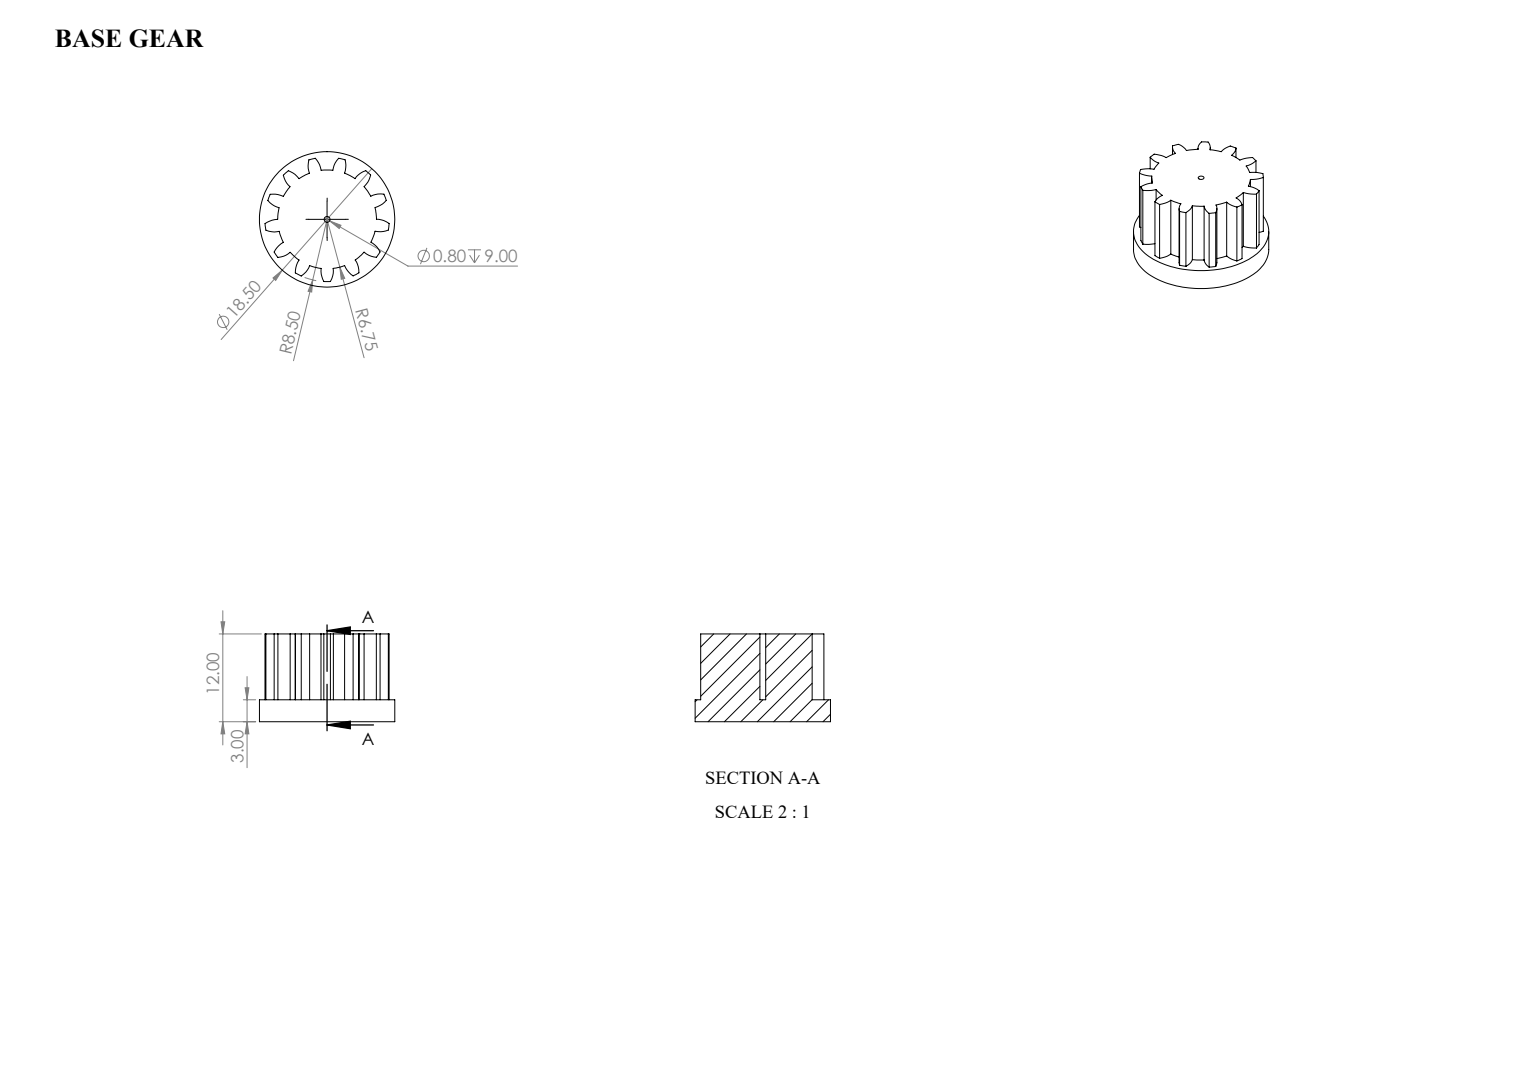
ISO-10303-21;
HEADER;
FILE_DESCRIPTION (('STEP AP214'),
    '1' );
FILE_NAME ('base-gear.step',
    '2026-10-11T23:18:24',
    ( '' ),
    ( '' ),
    'SwSTEP 2.0',
    'SolidWorks 2021',
    '' );
FILE_SCHEMA (( 'AUTOMOTIVE_DESIGN' ));
ENDSEC;

DATA;
#7=EDGE_CURVE ( 'NONE', #479, #8134, #9794, .T. ) ;
#20=VERTEX_POINT ( 'NONE', #10251 ) ;
#24=EDGE_CURVE ( 'NONE', #4332, #3918, #6675, .T. ) ;
#27=AXIS2_PLACEMENT_3D ( 'NONE', #4341, #12886, #6396 ) ;
#32=CARTESIAN_POINT ( 'NONE',  ( 2.458659560121117416, 9.000000000000000000, -8.136645080586040635 ) ) ;
#36=CARTESIAN_POINT ( 'NONE',  ( -3.835481108877868195, 0.000000000000000000, 5.554420281491219136 ) ) ;
#39=CYLINDRICAL_SURFACE ( 'NONE', #3345, 6.750000000000000888 ) ;
#44=EDGE_CURVE ( 'NONE', #672, #1296, #10164, .T. ) ;
#46=EDGE_LOOP ( 'NONE', ( #628, #4486, #10003, #7666 ) ) ;
#56=EDGE_LOOP ( 'NONE', ( #12824, #10379, #9147, #863 ) ) ;
#62=B_SPLINE_SURFACE_WITH_KNOTS ( 'NONE', 3, 1, ( 
 ( #3640, #12274 ),
 ( #3773, #7979 ),
 ( #12201, #7023 ),
 ( #11219, #1791 ) ),
 .UNSPECIFIED., .F., .F., .F.,
 ( 4, 4 ),
 ( 2, 2 ),
 ( 0.1276832474596304168, 1.000000000000000000 ),
 ( 0.000000000000000000, 1.000000000000000000 ),
 .UNSPECIFIED. ) ;
#70=DIRECTION ( 'NONE',  ( 0.000000000000000000, -1.000000000000000000, 0.000000000000000000 ) ) ;
#75=VERTEX_POINT ( 'NONE', #8304 ) ;
#76=VERTEX_POINT ( 'NONE', #2943 ) ;
#80=AXIS2_PLACEMENT_3D ( 'NONE', #518, #2715, #10017 ) ;
#87=CARTESIAN_POINT ( 'NONE',  ( -3.835481108877868195, 9.000000000000000000, 5.554420281491219136 ) ) ;
#100=ORIENTED_EDGE ( 'NONE', *, *, #3165, .F. ) ;
#101=VECTOR ( 'NONE', #278, 1000.000000000000000 ) ;
#108=EDGE_CURVE ( 'NONE', #3124, #12047, #7960, .T. ) ;
#114=PLANE ( 'NONE',  #5341 ) ;
#125=EDGE_CURVE ( 'NONE', #3742, #5918, #6114, .T. ) ;
#126=CARTESIAN_POINT ( 'NONE',  ( 7.659717769608228366, -1.694065894508600678E-18, -2.099897208369672530 ) ) ;
#136=CYLINDRICAL_SURFACE ( 'NONE', #4471, 8.499999999999996447 ) ;
#138=AXIS2_PLACEMENT_3D ( 'NONE', #9774, #352, #10185 ) ;
#141=EDGE_CURVE ( 'NONE', #20, #6815, #252, .T. ) ;
#154=PLANE ( 'NONE',  #12644 ) ;
#155=CARTESIAN_POINT ( 'NONE',  ( -7.155006492985575228, 0.000000000000000000, -1.740452503570284915 ) ) ;
#175=VERTEX_POINT ( 'NONE', #12924 ) ;
#182=CARTESIAN_POINT ( 'NONE',  ( 7.151505841916629080, 9.000000000000000000, 1.752496229622501511 ) ) ;
#183=CARTESIAN_POINT ( 'NONE',  ( 2.458659560121116527, 0.000000000000000000, -8.136645080586040635 ) ) ;
#184=CARTESIAN_POINT ( 'NONE',  ( -7.144272221052618832, 9.000000000000000000, 1.784003156764502940 ) ) ;
#187=CARTESIAN_POINT ( 'NONE',  ( 4.355042381134426321, 9.000000000000000000, 7.299562031966228659 ) ) ;
#188=ORIENTED_EDGE ( 'NONE', *, *, #12912, .F. ) ;
#191=ADVANCED_FACE ( 'NONE', ( #1279 ), #11366, .T. ) ;
#200=CARTESIAN_POINT ( 'NONE',  ( 0.000000000000000000, 0.000000000000000000, 0.000000000000000000 ) ) ;
#209=ORIENTED_EDGE ( 'NONE', *, *, #7248, .F. ) ;
#214=LINE ( 'NONE', #2474, #9546 ) ;
#220=EDGE_LOOP ( 'NONE', ( #4199, #4816, #462, #4259 ) ) ;
#221=VECTOR ( 'NONE', #9431, 1000.000000000000000 ) ;
#235=ORIENTED_EDGE ( 'NONE', *, *, #9698, .T. ) ;
#237=ORIENTED_EDGE ( 'NONE', *, *, #7398, .T. ) ;
#248=CARTESIAN_POINT ( 'NONE',  ( 0.4639228963249704130, 0.000000000000000000, 8.487330295579726069 ) ) ;
#252=LINE ( 'NONE', #10721, #2679 ) ;
#256=DIRECTION ( 'NONE',  ( -0.000000000000000000, -1.000000000000000000, -0.000000000000000000 ) ) ;
#258=CARTESIAN_POINT ( 'NONE',  ( 5.985774866078160450, 9.000000000000000000, 3.119775513178307147 ) ) ;
#262=B_SPLINE_SURFACE_WITH_KNOTS ( 'NONE', 3, 1, ( 
 ( #1876, #12212 ),
 ( #3923, #7034 ),
 ( #7178, #4068 ),
 ( #11374, #6196 ) ),
 .UNSPECIFIED., .F., .F., .F.,
 ( 4, 4 ),
 ( 2, 2 ),
 ( 0.1276832474596238665, 1.000000000000000000 ),
 ( 0.000000000000000000, 1.000000000000000000 ),
 .UNSPECIFIED. ) ;
#266=EDGE_LOOP ( 'NONE', ( #10134, #2477, #2333, #5399 ) ) ;
#278=DIRECTION ( 'NONE',  ( -0.000000000000000000, -1.000000000000000000, -0.000000000000000000 ) ) ;
#279=EDGE_CURVE ( 'NONE', #8354, #8278, #7045, .T. ) ;
#282=ORIENTED_EDGE ( 'NONE', *, *, #5312, .T. ) ;
#290=EDGE_CURVE ( 'NONE', #11016, #1998, #3872, .T. ) ;
#296=AXIS2_PLACEMENT_3D ( 'NONE', #2142, #10485, #1885 ) ;
#297=LINE ( 'NONE', #4418, #7104 ) ;
#301=EDGE_CURVE ( 'NONE', #13005, #4332, #5938, .T. ) ;
#318=VECTOR ( 'NONE', #11914, 1000.000000000000000 ) ;
#321=EDGE_CURVE ( 'NONE', #11737, #6548, #895, .T. ) ;
#328=ORIENTED_EDGE ( 'NONE', *, *, #3752, .F. ) ;
#338=CARTESIAN_POINT ( 'NONE',  ( 0.000000000000000000, 9.000000000000000000, 0.000000000000000000 ) ) ;
#339=ORIENTED_EDGE ( 'NONE', *, *, #792, .F. ) ;
#346=EDGE_CURVE ( 'NONE', #9464, #11924, #3340, .T. ) ;
#347=CARTESIAN_POINT ( 'NONE',  ( -8.369528376005813897, 9.000000000000000000, 1.483574994138650460 ) ) ;
#352=DIRECTION ( 'NONE',  ( 0.000000000000000000, 1.000000000000000000, -0.000000000000000000 ) ) ;
#363=EDGE_LOOP ( 'NONE', ( #4629, #4721, #6765, #6549 ) ) ;
#365=CYLINDRICAL_SURFACE ( 'NONE', #13589, 8.500000000000000000 ) ;
#368=CYLINDRICAL_SURFACE ( 'NONE', #6691, 6.749999999999999112 ) ;
#369=ADVANCED_FACE ( 'NONE', ( #11247 ), #1681, .T. ) ;
#373=CARTESIAN_POINT ( 'NONE',  ( 5.504794476853524188, 9.000000000000000000, -4.890042597913815570 ) ) ;
#378=CARTESIAN_POINT ( 'NONE',  ( -8.479748006907131597, 0.000000000000000000, 0.5864074857593127854 ) ) ;
#380=CARTESIAN_POINT ( 'NONE',  ( -7.144272221052618832, 0.000000000000000000, 1.784003156764502940 ) ) ;
#386=CARTESIAN_POINT ( 'NONE',  ( -2.655466033450426533, 9.000000000000000000, -7.485541762018160128 ) ) ;
#398=EDGE_LOOP ( 'NONE', ( #7206, #12127, #10777, #6516 ) ) ;
#400=ORIENTED_EDGE ( 'NONE', *, *, #9698, .F. ) ;
#404=DIRECTION ( 'NONE',  ( 0.000000000000000000, 0.000000000000000000, -1.000000000000000000 ) ) ;
#405=FACE_OUTER_BOUND ( 'NONE', #6501, .T. ) ;
#407=CARTESIAN_POINT ( 'NONE',  ( -5.065227977808753224, 9.000000000000000000, -4.461610195077944319 ) ) ;
#413=EDGE_CURVE ( 'NONE', #5612, #7910, #10086, .T. ) ;
#421=CARTESIAN_POINT ( 'NONE',  ( 0.8327827707325452522, 0.000000000000000000, 6.698430626405787791 ) ) ;
#427=EDGE_CURVE ( 'NONE', #11681, #3761, #12365, .T. ) ;
#434=VECTOR ( 'NONE', #1224, 1000.000000000000000 ) ;
#439=CARTESIAN_POINT ( 'NONE',  ( 7.363612555047485131, 0.000000000000000000, -0.02242701489043354146 ) ) ;
#440=LINE ( 'NONE', #7672, #4428 ) ;
#451=CARTESIAN_POINT ( 'NONE',  ( 0.000000000000000000, 9.000000000000000000, 0.000000000000000000 ) ) ;
#454=DIRECTION ( 'NONE',  ( 0.000000000000000000, 0.000000000000000000, 1.000000000000000000 ) ) ;
#456=LINE ( 'NONE', #4526, #902 ) ;
#460=EDGE_CURVE ( 'NONE', #8976, #10417, #11713, .T. ) ;
#462=ORIENTED_EDGE ( 'NONE', *, *, #10785, .F. ) ;
#476=DIRECTION ( 'NONE',  ( 0.000000000000000000, 0.000000000000000000, -1.000000000000000000 ) ) ;
#479=VERTEX_POINT ( 'NONE', #12756 ) ;
#490=EDGE_CURVE ( 'NONE', #10298, #5890, #7389, .T. ) ;
#504=AXIS2_PLACEMENT_3D ( 'NONE', #4653, #13064, #10988 ) ;
#510=EDGE_CURVE ( 'NONE', #12325, #8354, #13389, .T. ) ;
#514=CARTESIAN_POINT ( 'NONE',  ( 0.000000000000000000, 9.000000000000000000, 0.000000000000000000 ) ) ;
#518=CARTESIAN_POINT ( 'NONE',  ( 0.000000000000000000, 9.000000000000000000, 0.000000000000000000 ) ) ;
#529=AXIS2_PLACEMENT_3D ( 'NONE', #3588, #12216, #3653 ) ;
#533=CARTESIAN_POINT ( 'NONE',  ( 4.652003457867571967, 9.000000000000000000, -6.437678087145717321 ) ) ;
#535=EDGE_CURVE ( 'NONE', #8580, #8655, #4009, .T. ) ;
#539=AXIS2_PLACEMENT_3D ( 'NONE', #2331, #9566, #7561 ) ;
#540=DIRECTION ( 'NONE',  ( 0.000000000000000000, 1.000000000000000000, -0.000000000000000000 ) ) ;
#542=ORIENTED_EDGE ( 'NONE', *, *, #301, .T. ) ;
#558=CARTESIAN_POINT ( 'NONE',  ( 8.093005444143644311, 9.000000000000000000, -2.598704077239528232 ) ) ;
#564=ORIENTED_EDGE ( 'NONE', *, *, #7340, .T. ) ;
#569=FILL_AREA_STYLE ('',( #9990 ) ) ;
#573=FACE_OUTER_BOUND ( 'NONE', #5707, .T. ) ;
#586=CARTESIAN_POINT ( 'NONE',  ( 5.967832595844251742, 0.000000000000000000, -3.153961652902404822 ) ) ;
#591=DIRECTION ( 'NONE',  ( -0.000000000000000000, -1.000000000000000000, -0.000000000000000000 ) ) ;
#600=DIRECTION ( 'NONE',  ( 0.000000000000000000, 0.000000000000000000, 1.000000000000000000 ) ) ;
#609=EDGE_CURVE ( 'NONE', #5612, #2261, #8875, .T. ) ;
#613=EDGE_CURVE ( 'NONE', #1248, #75, #3577, .T. ) ;
#615=DIRECTION ( 'NONE',  ( 0.000000000000000000, 1.000000000000000000, -0.000000000000000000 ) ) ;
#628=ORIENTED_EDGE ( 'NONE', *, *, #460, .T. ) ;
#633=CARTESIAN_POINT ( 'NONE',  ( -5.830003112347290184, 0.000000000000000000, -5.394061460138155795 ) ) ;
#635=CARTESIAN_POINT ( 'NONE',  ( -0.8148820470561124463, 0.000000000000000000, 6.700631854488474204 ) ) ;
#640=ADVANCED_FACE ( 'NONE', ( #7783 ), #12001, .T. ) ;
#647=CARTESIAN_POINT ( 'NONE',  ( 0.000000000000000000, 9.000000000000000000, 0.000000000000000000 ) ) ;
#650=CARTESIAN_POINT ( 'NONE',  ( 8.373678438139048552, 9.000000000000000000, 1.459968977288628178 ) ) ;
#657=VECTOR ( 'NONE', #1576, 1000.000000000000000 ) ;
#658=ORIENTED_EDGE ( 'NONE', *, *, #13257, .F. ) ;
#663=CYLINDRICAL_SURFACE ( 'NONE', #1571, 6.749999999999999112 ) ;
#667=CARTESIAN_POINT ( 'NONE',  ( 7.248474140376191421, 9.000000000000000000, 4.439552076088042476 ) ) ;
#672=VERTEX_POINT ( 'NONE', #12826 ) ;
#676=DIRECTION ( 'NONE',  ( 0.000000000000000000, 0.000000000000000000, 1.000000000000000000 ) ) ;
#679=DIRECTION ( 'NONE',  ( -0.000000000000000000, -1.000000000000000000, -0.000000000000000000 ) ) ;
#703=CARTESIAN_POINT ( 'NONE',  ( -5.526615004551211463, 0.000000000000000000, -4.866191470063547797 ) ) ;
#706=LINE ( 'NONE', #11030, #6217 ) ;
#710=VERTEX_POINT ( 'NONE', #10194 ) ;
#711=DIRECTION ( 'NONE',  ( -0.000000000000000000, -1.000000000000000000, -0.000000000000000000 ) ) ;
#718=CARTESIAN_POINT ( 'NONE',  ( 0.000000000000000000, 0.000000000000000000, 0.000000000000000000 ) ) ;
#720=EDGE_CURVE ( 'NONE', #5890, #9922, #3343, .T. ) ;
#723=CARTESIAN_POINT ( 'NONE',  ( -5.299649803506881085, 0.000000000000000000, -6.645578376649351249 ) ) ;
#729=ORIENTED_EDGE ( 'NONE', *, *, #5793, .F. ) ;
#737=EDGE_CURVE ( 'NONE', #3503, #12047, #9277, .T. ) ;
#743=CARTESIAN_POINT ( 'NONE',  ( 7.771282357155270937, 9.000000000000000000, -3.443424244174282833 ) ) ;
#745=DIRECTION ( 'NONE',  ( 0.000000000000000000, 0.000000000000000000, 1.000000000000000000 ) ) ;
#747=ORIENTED_EDGE ( 'NONE', *, *, #4870, .F. ) ;
#752=AXIS2_PLACEMENT_3D ( 'NONE', #5759, #540, #3011 ) ;
#754=ORIENTED_EDGE ( 'NONE', *, *, #11345, .T. ) ;
#758=DIRECTION ( 'NONE',  ( -0.000000000000000000, -1.000000000000000000, -0.000000000000000000 ) ) ;
#759=CIRCLE ( 'NONE', #12438, 6.749999999999999112 ) ;
#762=CYLINDRICAL_SURFACE ( 'NONE', #11276, 8.500000000000001776 ) ;
#764=VECTOR ( 'NONE', #12228, 1000.000000000000000 ) ;
#765=ORIENTED_EDGE ( 'NONE', *, *, #1720, .F. ) ;
#766=CARTESIAN_POINT ( 'NONE',  ( 5.051606143860418285, 9.000000000000000000, 4.477027514692275112 ) ) ;
#767=EDGE_LOOP ( 'NONE', ( #4537, #1649, #2280, #9539 ) ) ;
#768=ORIENTED_EDGE ( 'NONE', *, *, #11051, .T. ) ;
#771=EDGE_LOOP ( 'NONE', ( #11809, #6157, #8797, #4003 ) ) ;
#778=CARTESIAN_POINT ( 'NONE',  ( -7.668956737359326148, 9.000000000000000000, -2.066866683227997825 ) ) ;
#789=ORIENTED_EDGE ( 'NONE', *, *, #10527, .F. ) ;
#792=EDGE_CURVE ( 'NONE', #11192, #8134, #10615, .T. ) ;
#813=CARTESIAN_POINT ( 'NONE',  ( 5.806472362263156661, -1.694065894508600678E-18, -5.419014975255640465 ) ) ;
#832=DIRECTION ( 'NONE',  ( 0.000000000000000000, 1.000000000000000000, -0.000000000000000000 ) ) ;
#863=ORIENTED_EDGE ( 'NONE', *, *, #8463, .T. ) ;
#893=ORIENTED_EDGE ( 'NONE', *, *, #8265, .T. ) ;
#895=B_SPLINE_CURVE_WITH_KNOTS ( 'NONE', 3,
 ( #4835, #5874, #2772, #9106 ),
 .UNSPECIFIED., .F., .F.,
 ( 4, 4 ),
 ( 0.1276832474596280298, 1.000000000000000000 ),
 .UNSPECIFIED. ) ;
#896=UNCERTAINTY_MEASURE_WITH_UNIT (LENGTH_MEASURE( 1.000000000000000082E-05 ), #12069, 'distance_accuracy_value', 'NONE');
#900=CARTESIAN_POINT ( 'NONE',  ( 2.392396671352951198, 0.000000000000000000, 6.311809420990095454 ) ) ;
#902=VECTOR ( 'NONE', #7758, 1000.000000000000000 ) ;
#904=CARTESIAN_POINT ( 'NONE',  ( -2.375523406013125616, 9.000000000000000000, 6.318179211409232998 ) ) ;
#910=CARTESIAN_POINT ( 'NONE',  ( 2.394769219159762041, 9.000000000000000000, -6.310909632292713844 ) ) ;
#912=VERTEX_POINT ( 'NONE', #8318 ) ;
#914=AXIS2_PLACEMENT_3D ( 'NONE', #6046, #5067, #11412 ) ;
#915=AXIS2_PLACEMENT_3D ( 'NONE', #514, #12237, #8971 ) ;
#918=CARTESIAN_POINT ( 'NONE',  ( -1.161309641800940540, 9.000000000000000000, -7.856984441350959969 ) ) ;
#919=CARTESIAN_POINT ( 'NONE',  ( -6.721397655168936502, 0.000000000000000000, 5.203154193476255074 ) ) ;
#920=CARTESIAN_POINT ( 'NONE',  ( 2.394769219159762930, 0.000000000000000000, -6.310909632292713844 ) ) ;
#924=VECTOR ( 'NONE', #7658, 1000.000000000000000 ) ;
#929=CARTESIAN_POINT ( 'NONE',  ( -7.751044794789887504, 9.000000000000000000, 1.733822342365972879 ) ) ;
#933=VERTEX_POINT ( 'NONE', #4262 ) ;
#934=CIRCLE ( 'NONE', #10828, 6.750000000000000888 ) ;
#941=DIRECTION ( 'NONE',  ( 0.000000000000000000, 0.000000000000000000, 1.000000000000000000 ) ) ;
#945=DIRECTION ( 'NONE',  ( 0.000000000000000000, 1.000000000000000000, -0.000000000000000000 ) ) ;
#952=AXIS2_PLACEMENT_3D ( 'NONE', #7370, #1092, #8383 ) ;
#960=CARTESIAN_POINT ( 'NONE',  ( 0.000000000000000000, 9.000000000000000000, 0.000000000000000000 ) ) ;
#965=CIRCLE ( 'NONE', #752, 0.4000000000000000222 ) ;
#969=EDGE_CURVE ( 'NONE', #12363, #7708, #11509, .T. ) ;
#984=CARTESIAN_POINT ( 'NONE',  ( 2.601737331980797041, 9.000000000000000000, -6.888123234756056590 ) ) ;
#989=CARTESIAN_POINT ( 'NONE',  ( 0.000000000000000000, 9.000000000000000000, 0.000000000000000000 ) ) ;
#1004=VERTEX_POINT ( 'NONE', #8188 ) ;
#1018=DIRECTION ( 'NONE',  ( 0.000000000000000000, 0.000000000000000000, -1.000000000000000000 ) ) ;
#1022=LINE ( 'NONE', #9481, #434 ) ;
#1024=FACE_BOUND ( 'NONE', #7694, .T. ) ;
#1038=DIRECTION ( 'NONE',  ( -0.000000000000000000, 1.000000000000000000, -0.000000000000000000 ) ) ;
#1047=ORIENTED_EDGE ( 'NONE', *, *, #6279, .F. ) ;
#1050=ORIENTED_EDGE ( 'NONE', *, *, #6088, .F. ) ;
#1056=CARTESIAN_POINT ( 'NONE',  ( -6.524296280129988190, 0.000000000000000000, -3.413039245436654490 ) ) ;
#1057=EDGE_CURVE ( 'NONE', #8876, #11924, #1835, .T. ) ;
#1062=FACE_OUTER_BOUND ( 'NONE', #6446, .T. ) ;
#1068=ORIENTED_EDGE ( 'NONE', *, *, #2402, .F. ) ;
#1076=ORIENTED_EDGE ( 'NONE', *, *, #125, .T. ) ;
#1079=CARTESIAN_POINT ( 'NONE',  ( -3.833392836528144443, 9.000000000000000000, -5.555861711818853799 ) ) ;
#1092=DIRECTION ( 'NONE',  ( 0.000000000000000000, 1.000000000000000000, -0.000000000000000000 ) ) ;
#1097=CARTESIAN_POINT ( 'NONE',  ( -6.934601996837493232, 9.000000000000000000, 3.871968458191308748 ) ) ;
#1123=CARTESIAN_POINT ( 'NONE',  ( 3.818534268238711782, 0.000000000000000000, -5.566084444408534004 ) ) ;
#1125=FACE_OUTER_BOUND ( 'NONE', #10996, .T. ) ;
#1135=CARTESIAN_POINT ( 'NONE',  ( 4.369710415961185035, 0.000000000000000000, 6.632530905044255576 ) ) ;
#1152=AXIS2_PLACEMENT_3D ( 'NONE', #10267, #11093, #13302 ) ;
#1155=DIRECTION ( 'NONE',  ( 0.000000000000000000, 1.000000000000000000, -0.000000000000000000 ) ) ;
#1159=VERTEX_POINT ( 'NONE', #4600 ) ;
#1172=DIRECTION ( 'NONE',  ( 0.000000000000000000, 1.000000000000000000, -0.000000000000000000 ) ) ;
#1177=CARTESIAN_POINT ( 'NONE',  ( -2.375523406013128280, 0.000000000000000000, 6.318179211409232998 ) ) ;
#1181=ORIENTED_EDGE ( 'NONE', *, *, #11088, .T. ) ;
#1182=ORIENTED_EDGE ( 'NONE', *, *, #3026, .T. ) ;
#1192=CARTESIAN_POINT ( 'NONE',  ( 0.000000000000000000, 0.000000000000000000, -0.4000000000000000222 ) ) ;
#1194=LINE ( 'NONE', #10898, #1407 ) ;
#1205=ORIENTED_EDGE ( 'NONE', *, *, #12589, .F. ) ;
#1208=LINE ( 'NONE', #5332, #2944 ) ;
#1212=CARTESIAN_POINT ( 'NONE',  ( -7.939678587550617728, 9.000000000000000000, 0.2057875656132798770 ) ) ;
#1216=ADVANCED_FACE ( 'NONE', ( #10172 ), #3764, .T. ) ;
#1224=DIRECTION ( 'NONE',  ( -0.000000000000000000, -1.000000000000000000, -0.000000000000000000 ) ) ;
#1241=CARTESIAN_POINT ( 'NONE',  ( 5.051606143860418285, 1.734723475976807094E-15, 4.477027514692275112 ) ) ;
#1243=CARTESIAN_POINT ( 'NONE',  ( -5.039625798601655937, 9.000000000000000000, 4.490509081392509927 ) ) ;
#1248=VERTEX_POINT ( 'NONE', #6868 ) ;
#1255=CARTESIAN_POINT ( 'NONE',  ( -5.975392301194330180, 9.000000000000000000, -6.045220165289885372 ) ) ;
#1267=CARTESIAN_POINT ( 'NONE',  ( -0.7527353566742582824, 9.000000000000000000, 7.906594341344654886 ) ) ;
#1276=EDGE_CURVE ( 'NONE', #2790, #9600, #6442, .T. ) ;
#1279=FACE_OUTER_BOUND ( 'NONE', #4502, .T. ) ;
#1284=DIRECTION ( 'NONE',  ( 0.000000000000000000, -0.000000000000000000, -1.000000000000000000 ) ) ;
#1287=CARTESIAN_POINT ( 'NONE',  ( 8.373678438139048552, 9.000000000000000000, 1.459968977288628178 ) ) ;
#1292=ORIENTED_EDGE ( 'NONE', *, *, #7345, .T. ) ;
#1296=VERTEX_POINT ( 'NONE', #7830 ) ;
#1301=DIRECTION ( 'NONE',  ( 0.000000000000000000, 0.000000000000000000, 1.000000000000000000 ) ) ;
#1304=CARTESIAN_POINT ( 'NONE',  ( 0.000000000000000000, 9.000000000000000000, 0.000000000000000000 ) ) ;
#1321=DIRECTION ( 'NONE',  ( -0.000000000000000000, -1.000000000000000000, -0.000000000000000000 ) ) ;
#1324=ORIENTED_EDGE ( 'NONE', *, *, #13353, .T. ) ;
#1328=ADVANCED_FACE ( 'NONE', ( #9353 ), #3014, .T. ) ;
#1329=ORIENTED_EDGE ( 'NONE', *, *, #4134, .T. ) ;
#1330=CARTESIAN_POINT ( 'NONE',  ( -0.8148820470561131124, 9.000000000000000000, 6.700631854488474204 ) ) ;
#1337=B_SPLINE_CURVE_WITH_KNOTS ( 'NONE', 3,
 ( #8936, #4809, #13213, #2810 ),
 .UNSPECIFIED., .F., .F.,
 ( 4, 4 ),
 ( 0.1276832474596304168, 1.000000000000000000 ),
 .UNSPECIFIED. ) ;
#1341=CARTESIAN_POINT ( 'NONE',  ( 3.850308450823737960, 0.000000000000000000, 5.544152309732778505 ) ) ;
#1343=EDGE_CURVE ( 'NONE', #1554, #7708, #11723, .T. ) ;
#1344=CIRCLE ( 'NONE', #914, 8.500000000000000000 ) ;
#1349=B_SPLINE_CURVE_WITH_KNOTS ( 'NONE', 3,
 ( #8865, #2672, #3771, #9974 ),
 .UNSPECIFIED., .F., .F.,
 ( 4, 4 ),
 ( 0.1276832474596248101, 1.000000000000000000 ),
 .UNSPECIFIED. ) ;
#1350=CARTESIAN_POINT ( 'NONE',  ( 7.110882674384088276, 0.000000000000000000, -3.538387050178523729 ) ) ;
#1353=DIRECTION ( 'NONE',  ( -0.000000000000000000, -1.000000000000000000, -0.000000000000000000 ) ) ;
#1354=DIRECTION ( 'NONE',  ( -0.000000000000000000, -1.000000000000000000, -0.000000000000000000 ) ) ;
#1368=CARTESIAN_POINT ( 'NONE',  ( 0.000000000000000000, 9.000000000000000000, 0.000000000000000000 ) ) ;
#1377=VECTOR ( 'NONE', #711, 1000.000000000000000 ) ;
#1379=AXIS2_PLACEMENT_3D ( 'NONE', #6970, #9916, #13027 ) ;
#1386=ORIENTED_EDGE ( 'NONE', *, *, #11832, .T. ) ;
#1397=CARTESIAN_POINT ( 'NONE',  ( -0.8776997859584816375, 0.000000000000000000, 7.310603390113379341 ) ) ;
#1407=VECTOR ( 'NONE', #12704, 1000.000000000000000 ) ;
#1413=CARTESIAN_POINT ( 'NONE',  ( 8.481367827640703183, 9.000000000000000000, 0.5624942419805130100 ) ) ;
#1429=CARTESIAN_POINT ( 'NONE',  ( 1.580708947611199511, 0.000000000000000000, -8.351727918397596540 ) ) ;
#1438=ORIENTED_EDGE ( 'NONE', *, *, #4998, .F. ) ;
#1444=CARTESIAN_POINT ( 'NONE',  ( -4.334442004268530546, 9.000000000000000000, 7.311813216407585081 ) ) ;
#1446=CARTESIAN_POINT ( 'NONE',  ( 0.000000000000000000, 9.000000000000000000, 0.000000000000000000 ) ) ;
#1448=CARTESIAN_POINT ( 'NONE',  ( -8.479748006907131597, 0.000000000000000000, 0.5864074857593127854 ) ) ;
#1458=ORIENTED_EDGE ( 'NONE', *, *, #8658, .F. ) ;
#1461=ORIENTED_EDGE ( 'NONE', *, *, #11441, .T. ) ;
#1462=LINE ( 'NONE', #12068, #9122 ) ;
#1466=CARTESIAN_POINT ( 'NONE',  ( 0.9098489087730803337, 9.000000000000000000, 7.307220250892556557 ) ) ;
#1473=ORIENTED_EDGE ( 'NONE', *, *, #141, .T. ) ;
#1478=EDGE_CURVE ( 'NONE', #2415, #12329, #10151, .T. ) ;
#1483=CARTESIAN_POINT ( 'NONE',  ( 0.000000000000000000, 9.000000000000000000, 0.000000000000000000 ) ) ;
#1485=ORIENTED_EDGE ( 'NONE', *, *, #10916, .T. ) ;
#1494=CARTESIAN_POINT ( 'NONE',  ( -7.235926821844430812, 9.000000000000000000, 4.459973433655439301 ) ) ;
#1495=B_SPLINE_CURVE_WITH_KNOTS ( 'NONE', 3,
 ( #378, #6768, #3806, #3599 ),
 .UNSPECIFIED., .F., .F.,
 ( 4, 4 ),
 ( 0.1276832474596284739, 1.000000000000000000 ),
 .UNSPECIFIED. ) ;
#1497=DIRECTION ( 'NONE',  ( -0.000000000000000000, -1.000000000000000000, -0.000000000000000000 ) ) ;
#1509=CARTESIAN_POINT ( 'NONE',  ( 5.967832595844252630, 0.000000000000000000, -3.153961652902406154 ) ) ;
#1514=DIRECTION ( 'NONE',  ( 0.000000000000000000, 0.000000000000000000, -1.000000000000000000 ) ) ;
#1516=ORIENTED_EDGE ( 'NONE', *, *, #12315, .T. ) ;
#1522=EDGE_CURVE ( 'NONE', #7238, #10060, #4127, .T. ) ;
#1535=VERTEX_POINT ( 'NONE', #5152 ) ;
#1540=CARTESIAN_POINT ( 'NONE',  ( 4.355042381134428098, 0.000000000000000000, 7.299562031966232212 ) ) ;
#1544=CARTESIAN_POINT ( 'NONE',  ( 6.951477219042924816, 0.000000000000000000, 3.842108769784387423 ) ) ;
#1548=FACE_OUTER_BOUND ( 'NONE', #9846, .T. ) ;
#1554=VERTEX_POINT ( 'NONE', #11563 ) ;
#1555=EDGE_CURVE ( 'NONE', #12329, #2013, #3150, .T. ) ;
#1565=CARTESIAN_POINT ( 'NONE',  ( 0.4639228963249696913, 9.000000000000000000, 8.487330295579727846 ) ) ;
#1571=AXIS2_PLACEMENT_3D ( 'NONE', #1768, #5267, #11551 ) ;
#1576=DIRECTION ( 'NONE',  ( -0.000000000000000000, -1.000000000000000000, -0.000000000000000000 ) ) ;
#1580=CARTESIAN_POINT ( 'NONE',  ( -5.975392301194330180, 9.000000000000000000, -6.045220165289885372 ) ) ;
#1581=CARTESIAN_POINT ( 'NONE',  ( 0.000000000000000000, 0.000000000000000000, 0.000000000000000000 ) ) ;
#1599=CIRCLE ( 'NONE', #4671, 6.750000000000000888 ) ;
#1604=ORIENTED_EDGE ( 'NONE', *, *, #11034, .F. ) ;
#1625=CARTESIAN_POINT ( 'NONE',  ( -8.479748006907131597, 9.000000000000000000, 0.5864074857593127854 ) ) ;
#1635=VECTOR ( 'NONE', #8325, 1000.000000000000000 ) ;
#1639=CARTESIAN_POINT ( 'NONE',  ( 0.8327827707325454742, 0.000000000000000000, 6.698430626405788679 ) ) ;
#1643=CIRCLE ( 'NONE', #10868, 8.499999999999996447 ) ;
#1649=ORIENTED_EDGE ( 'NONE', *, *, #10971, .F. ) ;
#1657=CARTESIAN_POINT ( 'NONE',  ( -6.721397655168936502, 9.000000000000000000, 5.203154193476255074 ) ) ;
#1658=CARTESIAN_POINT ( 'NONE',  ( -5.526615004551211463, 9.000000000000000000, -4.866191470063547797 ) ) ;
#1660=DIRECTION ( 'NONE',  ( -0.000000000000000000, -1.000000000000000000, -0.000000000000000000 ) ) ;
#1672=CARTESIAN_POINT ( 'NONE',  ( -5.975392301194336397, 0.000000000000000000, -6.045220165289885372 ) ) ;
#1681=CYLINDRICAL_SURFACE ( 'NONE', #6432, 8.499999999999998224 ) ;
#1685=ADVANCED_FACE ( 'NONE', ( #11623 ), #136, .T. ) ;
#1686=DIRECTION ( 'NONE',  ( -0.000000000000000000, -1.000000000000000000, -0.000000000000000000 ) ) ;
#1689=CARTESIAN_POINT ( 'NONE',  ( -3.833392836528145331, 0.000000000000000000, -5.555861711818853799 ) ) ;
#1691=CARTESIAN_POINT ( 'NONE',  ( 0.4639228963249696913, 9.000000000000000000, 8.487330295579727846 ) ) ;
#1698=EDGE_CURVE ( 'NONE', #12325, #5342, #9679, .T. ) ;
#1706=FACE_OUTER_BOUND ( 'NONE', #9694, .T. ) ;
#1708=CARTESIAN_POINT ( 'NONE',  ( 6.530577460941774603, 9.000000000000000000, 3.402183248810843885 ) ) ;
#1711=ORIENTED_EDGE ( 'NONE', *, *, #413, .T. ) ;
#1712=B_SPLINE_SURFACE_WITH_KNOTS ( 'NONE', 3, 1, ( 
 ( #8387, #10606 ),
 ( #1097, #5174 ),
 ( #9497, #12614 ),
 ( #11581, #4338 ) ),
 .UNSPECIFIED., .F., .F., .F.,
 ( 4, 4 ),
 ( 2, 2 ),
 ( 0.1276832474596353850, 1.000000000000000000 ),
 ( 0.000000000000000000, 1.000000000000000000 ),
 .UNSPECIFIED. ) ;
#1720=EDGE_CURVE ( 'NONE', #11943, #175, #2501, .T. ) ;
#1750=CARTESIAN_POINT ( 'NONE',  ( -5.039625798601655937, 0.000000000000000000, 4.490509081392509927 ) ) ;
#1763=ORIENTED_EDGE ( 'NONE', *, *, #5633, .F. ) ;
#1768=CARTESIAN_POINT ( 'NONE',  ( 0.000000000000000000, 9.000000000000000000, 0.000000000000000000 ) ) ;
#1776=EDGE_LOOP ( 'NONE', ( #8565, #9760, #5526, #11107 ) ) ;
#1782=CARTESIAN_POINT ( 'NONE',  ( -6.721397655168936502, 0.000000000000000000, 5.203154193476255074 ) ) ;
#1791=CARTESIAN_POINT ( 'NONE',  ( -0.8123631076467130452, 0.000000000000000000, -6.700937709107178009 ) ) ;
#1792=ORIENTED_EDGE ( 'NONE', *, *, #969, .F. ) ;
#1796=EDGE_CURVE ( 'NONE', #7728, #11178, #3583, .T. ) ;
#1808=CARTESIAN_POINT ( 'NONE',  ( 1.580708947611198623, 9.000000000000000000, -8.351727918397600092 ) ) ;
#1815=VERTEX_POINT ( 'NONE', #5826 ) ;
#1818=CARTESIAN_POINT ( 'NONE',  ( 0.000000000000000000, 9.000000000000000000, 0.000000000000000000 ) ) ;
#1819=VECTOR ( 'NONE', #9647, 1000.000000000000000 ) ;
#1823=DIRECTION ( 'NONE',  ( 0.000000000000000000, 0.000000000000000000, 1.000000000000000000 ) ) ;
#1825=B_SPLINE_CURVE_WITH_KNOTS ( 'NONE', 3,
 ( #12649, #2229, #6436, #10647 ),
 .UNSPECIFIED., .F., .F.,
 ( 4, 4 ),
 ( 0.1276832474596353850, 1.000000000000000000 ),
 .UNSPECIFIED. ) ;
#1835=CIRCLE ( 'NONE', #4026, 6.749999999999999112 ) ;
#1851=CARTESIAN_POINT ( 'NONE',  ( 4.201465772524378472, 9.000000000000000000, 6.047394330962382547 ) ) ;
#1857=CARTESIAN_POINT ( 'NONE',  ( -3.533475733155565290, 9.000000000000000000, 7.730753471893975437 ) ) ;
#1865=DIRECTION ( 'NONE',  ( 0.000000000000000000, 1.000000000000000000, -0.000000000000000000 ) ) ;
#1869=ORIENTED_EDGE ( 'NONE', *, *, #6836, .F. ) ;
#1873=CIRCLE ( 'NONE', #7153, 6.750000000000000888 ) ;
#1876=CARTESIAN_POINT ( 'NONE',  ( 3.555260608155775159, 9.000000000000000000, 7.720759160088846329 ) ) ;
#1882=CARTESIAN_POINT ( 'NONE',  ( 3.555260608155774271, 0.000000000000000000, 7.720759160088842776 ) ) ;
#1885=DIRECTION ( 'NONE',  ( 0.000000000000000000, 0.000000000000000000, 1.000000000000000000 ) ) ;
#1889=CARTESIAN_POINT ( 'NONE',  ( -4.340891659662447388, -1.694065894508600678E-18, 6.651128039276029469 ) ) ;
#1892=CARTESIAN_POINT ( 'NONE',  ( -6.558450276537426404, 9.000000000000000000, -1.596630818375423866 ) ) ;
#1906=ORIENTED_EDGE ( 'NONE', *, *, #3581, .T. ) ;
#1937=CARTESIAN_POINT ( 'NONE',  ( 0.000000000000000000, 0.000000000000000000, 0.000000000000000000 ) ) ;
#1940=CARTESIAN_POINT ( 'NONE',  ( 0.7868956173019259204, 0.000000000000000000, 7.903520140620750034 ) ) ;
#1949=EDGE_LOOP ( 'NONE', ( #12098, #12630, #4544, #1473 ) ) ;
#1953=DIRECTION ( 'NONE',  ( 0.000000000000000000, 0.000000000000000000, 1.000000000000000000 ) ) ;
#1954=( LENGTH_UNIT ( ) NAMED_UNIT ( * ) SI_UNIT ( .MILLI., .METRE. ) );
#1959=CARTESIAN_POINT ( 'NONE',  ( -8.100301009650799244, 0.000000000000000000, -2.575873357339268033 ) ) ;
#1960=CARTESIAN_POINT ( 'NONE',  ( -4.334442004268525217, 0.000000000000000000, 7.311813216407587745 ) ) ;
#1965=ORIENTED_EDGE ( 'NONE', *, *, #9188, .F. ) ;
#1981=DIRECTION ( 'NONE',  ( 0.000000000000000000, 0.000000000000000000, 1.000000000000000000 ) ) ;
#1984=AXIS2_PLACEMENT_3D ( 'NONE', #12867, #3620, #9956 ) ;
#1990=DIRECTION ( 'NONE',  ( 0.000000000000000000, 0.000000000000000000, 1.000000000000000000 ) ) ;
#1998=VERTEX_POINT ( 'NONE', #4031 ) ;
#2011=CARTESIAN_POINT ( 'NONE',  ( 2.394769219159762930, 1.734723475976807094E-15, -6.310909632292713844 ) ) ;
#2013=VERTEX_POINT ( 'NONE', #11469 ) ;
#2017=ORIENTED_EDGE ( 'NONE', *, *, #12673, .F. ) ;
#2023=CARTESIAN_POINT ( 'NONE',  ( -2.411622991978541464, 9.000000000000000000, -6.304488444319688689 ) ) ;
#2030=DIRECTION ( 'NONE',  ( -0.000000000000000000, -1.000000000000000000, -0.000000000000000000 ) ) ;
#2048=ORIENTED_EDGE ( 'NONE', *, *, #108, .T. ) ;
#2049=CARTESIAN_POINT ( 'NONE',  ( -7.144272221052618832, 0.000000000000000000, 1.784003156764502940 ) ) ;
#2056=SHAPE_DEFINITION_REPRESENTATION ( #6336, #8376 ) ;
#2081=CARTESIAN_POINT ( 'NONE',  ( -2.481593227817850966, 0.000000000000000000, -8.129679886173169834 ) ) ;
#2093=CARTESIAN_POINT ( 'NONE',  ( -6.524296280129988190, 9.000000000000000000, -3.413039245436654490 ) ) ;
#2096=CARTESIAN_POINT ( 'NONE',  ( 5.051606143860418285, 1.734723475976807094E-15, 4.477027514692275112 ) ) ;
#2115=ADVANCED_FACE ( 'NONE', ( #7539 ), #11890, .T. ) ;
#2119=EDGE_CURVE ( 'NONE', #8226, #8945, #9223, .T. ) ;
#2128=ORIENTED_EDGE ( 'NONE', *, *, #2703, .T. ) ;
#2132=ORIENTED_EDGE ( 'NONE', *, *, #8959, .T. ) ;
#2136=CARTESIAN_POINT ( 'NONE',  ( 6.554160776451332104, 1.734723475976807094E-15, -1.614148852004323231 ) ) ;
#2139=CARTESIAN_POINT ( 'NONE',  ( 0.000000000000000000, 9.000000000000000000, 0.000000000000000000 ) ) ;
#2142=CARTESIAN_POINT ( 'NONE',  ( 0.000000000000000000, 0.000000000000000000, 0.000000000000000000 ) ) ;
#2147=CARTESIAN_POINT ( 'NONE',  ( 2.623034112301249721, 9.000000000000000000, -7.496701717520498853 ) ) ;
#2159=DIRECTION ( 'NONE',  ( 0.000000000000000000, 1.000000000000000000, -0.000000000000000000 ) ) ;
#2161=DIRECTION ( 'NONE',  ( 0.000000000000000000, 0.000000000000000000, -1.000000000000000000 ) ) ;
#2172=EDGE_CURVE ( 'NONE', #7190, #10761, #1208, .T. ) ;
#2178=ORIENTED_EDGE ( 'NONE', *, *, #6674, .T. ) ;
#2184=EDGE_CURVE ( 'NONE', #11220, #1535, #10650, .T. ) ;
#2186=DIRECTION ( 'NONE',  ( 0.000000000000000000, 0.000000000000000000, 1.000000000000000000 ) ) ;
#2195=CYLINDRICAL_SURFACE ( 'NONE', #9895, 9.250000000000000000 ) ;
#2196=EDGE_CURVE ( 'NONE', #12802, #20, #1825, .T. ) ;
#2197=LINE ( 'NONE', #87, #101 ) ;
#2207=EDGE_CURVE ( 'NONE', #10329, #13219, #6735, .T. ) ;
#2213=AXIS2_PLACEMENT_3D ( 'NONE', #2878, #758, #8114 ) ;
#2214=AXIS2_PLACEMENT_3D ( 'NONE', #12601, #70, #1284 ) ;
#2223=ORIENTED_EDGE ( 'NONE', *, *, #346, .F. ) ;
#2224=CARTESIAN_POINT ( 'NONE',  ( 5.958322434183389582, 9.000000000000000000, -6.062045345451230638 ) ) ;
#2225=AXIS2_PLACEMENT_3D ( 'NONE', #10092, #2795, #11271 ) ;
#2229=CARTESIAN_POINT ( 'NONE',  ( -6.934601996837493232, 9.000000000000000000, 3.871968458191308748 ) ) ;
#2232=EDGE_CURVE ( 'NONE', #7353, #5239, #8757, .T. ) ;
#2243=CARTESIAN_POINT ( 'NONE',  ( 0.000000000000000000, 9.000000000000000000, 0.000000000000000000 ) ) ;
#2245=VECTOR ( 'NONE', #9815, 1000.000000000000000 ) ;
#2252=CARTESIAN_POINT ( 'NONE',  ( 3.818534268238711782, 0.000000000000000000, -5.566084444408534004 ) ) ;
#2261=VERTEX_POINT ( 'NONE', #11947 ) ;
#2263=DIRECTION ( 'NONE',  ( 0.000000000000000000, 1.000000000000000000, -0.000000000000000000 ) ) ;
#2269=AXIS2_PLACEMENT_3D ( 'NONE', #12185, #1497, #12999 ) ;
#2272=AXIS2_PLACEMENT_3D ( 'NONE', #8521, #6469, #9573 ) ;
#2273=ORIENTED_EDGE ( 'NONE', *, *, #10801, .F. ) ;
#2280=ORIENTED_EDGE ( 'NONE', *, *, #10025, .F. ) ;
#2285=EDGE_CURVE ( 'NONE', #3746, #10516, #3395, .T. ) ;
#2300=EDGE_LOOP ( 'NONE', ( #3209, #7876, #1458, #4515 ) ) ;
#2302=EDGE_CURVE ( 'NONE', #11220, #9600, #5274, .T. ) ;
#2310=EDGE_CURVE ( 'NONE', #5342, #5243, #4489, .T. ) ;
#2320=EDGE_CURVE ( 'NONE', #11192, #5918, #1495, .T. ) ;
#2321=CARTESIAN_POINT ( 'NONE',  ( 3.850308450823737960, 9.000000000000000000, 5.544152309732778505 ) ) ;
#2322=EDGE_CURVE ( 'NONE', #8945, #6374, #9032, .T. ) ;
#2324=EDGE_LOOP ( 'NONE', ( #8109, #5994, #3687, #3675 ) ) ;
#2331=CARTESIAN_POINT ( 'NONE',  ( 0.000000000000000000, 0.000000000000000000, 0.000000000000000000 ) ) ;
#2333=ORIENTED_EDGE ( 'NONE', *, *, #10801, .T. ) ;
#2348=CARTESIAN_POINT ( 'NONE',  ( 7.940744365623959133, 9.000000000000000000, 0.1715058177969961128 ) ) ;
#2357=( LENGTH_UNIT ( ) NAMED_UNIT ( * ) SI_UNIT ( .MILLI., .METRE. ) );
#2372=CARTESIAN_POINT ( 'NONE',  ( 7.758214145541979967, 9.000000000000000000, 1.700281702449083054 ) ) ;
#2373=CARTESIAN_POINT ( 'NONE',  ( 8.481367827640703183, 0.000000000000000000, 0.5624942419805130100 ) ) ;
#2374=EDGE_CURVE ( 'NONE', #2415, #3742, #4270, .T. ) ;
#2384=ORIENTED_EDGE ( 'NONE', *, *, #12315, .F. ) ;
#2393=CYLINDRICAL_SURFACE ( 'NONE', #4693, 6.750000000000000888 ) ;
#2402=EDGE_CURVE ( 'NONE', #1248, #11926, #8062, .T. ) ;
#2403=CARTESIAN_POINT ( 'NONE',  ( 7.659717769608228366, 0.000000000000000000, -2.099897208369672530 ) ) ;
#2405=LINE ( 'NONE', #7381, #12593 ) ;
#2407=B_SPLINE_CURVE_WITH_KNOTS ( 'NONE', 3,
 ( #2626, #6826, #10133, #6901 ),
 .UNSPECIFIED., .F., .F.,
 ( 4, 4 ),
 ( 0.1276832474596250877, 1.000000000000000000 ),
 .UNSPECIFIED. ) ;
#2414=ORIENTED_EDGE ( 'NONE', *, *, #7339, .T. ) ;
#2415=VERTEX_POINT ( 'NONE', #1892 ) ;
#2432=CARTESIAN_POINT ( 'NONE',  ( 6.553553527263006551, 0.000000000000000000, 1.616612558808879774 ) ) ;
#2436=DIRECTION ( 'NONE',  ( 0.000000000000000000, 1.000000000000000000, -0.000000000000000000 ) ) ;
#2437=VECTOR ( 'NONE', #10525, 1000.000000000000000 ) ;
#2439=DIRECTION ( 'NONE',  ( -0.000000000000000000, -1.000000000000000000, -0.000000000000000000 ) ) ;
#2451=ADVANCED_FACE ( 'NONE', ( #8079 ), #4145, .T. ) ;
#2467=CIRCLE ( 'NONE', #12394, 8.499999999999996447 ) ;
#2474=CARTESIAN_POINT ( 'NONE',  ( 0.8327827707325454742, 9.000000000000000000, 6.698430626405788679 ) ) ;
#2477=ORIENTED_EDGE ( 'NONE', *, *, #1478, .F. ) ;
#2479=AXIS2_PLACEMENT_3D ( 'NONE', #11242, #9024, #4832 ) ;
#2480=ORIENTED_EDGE ( 'NONE', *, *, #6620, .F. ) ;
#2491=CIRCLE ( 'NONE', #10190, 8.499999999999998224 ) ;
#2493=CARTESIAN_POINT ( 'NONE',  ( 0.8327827707325452522, 9.000000000000000000, 6.698430626405787791 ) ) ;
#2494=AXIS2_PLACEMENT_3D ( 'NONE', #13026, #4690, #10061 ) ;
#2496=CARTESIAN_POINT ( 'NONE',  ( -5.830003112347290184, 0.000000000000000000, -5.394061460138155795 ) ) ;
#2499=CARTESIAN_POINT ( 'NONE',  ( 3.007863545083557355, 9.000000000000000000, 7.350755164602351677 ) ) ;
#2500=ORIENTED_EDGE ( 'NONE', *, *, #11734, .T. ) ;
#2501=CIRCLE ( 'NONE', #8427, 6.750000000000000888 ) ;
#2506=CARTESIAN_POINT ( 'NONE',  ( -0.8148820470561131124, 9.000000000000000000, 6.700631854488474204 ) ) ;
#2528=CARTESIAN_POINT ( 'NONE',  ( 6.951477219042924816, 9.000000000000000000, 3.842108769784387423 ) ) ;
#2532=EDGE_CURVE ( 'NONE', #10516, #3746, #4067, .T. ) ;
#2548=DIRECTION ( 'NONE',  ( 0.000000000000000000, 0.000000000000000000, 1.000000000000000000 ) ) ;
#2560=CARTESIAN_POINT ( 'NONE',  ( 1.580708947611199511, 9.000000000000000000, -8.351727918397596540 ) ) ;
#2561=( NAMED_UNIT ( * ) SI_UNIT ( $, .STERADIAN. ) SOLID_ANGLE_UNIT ( ) );
#2571=ORIENTED_EDGE ( 'NONE', *, *, #7250, .T. ) ;
#2586=ORIENTED_EDGE ( 'NONE', *, *, #279, .T. ) ;
#2588=DIRECTION ( 'NONE',  ( 0.000000000000000000, 1.000000000000000000, -0.000000000000000000 ) ) ;
#2594=CARTESIAN_POINT ( 'NONE',  ( -0.8148820470561131124, 9.000000000000000000, 6.700631854488474204 ) ) ;
#2595=ORIENTED_EDGE ( 'NONE', *, *, #609, .T. ) ;
#2603=DIRECTION ( 'NONE',  ( 0.000000000000000000, 1.000000000000000000, -0.000000000000000000 ) ) ;
#2604=CARTESIAN_POINT ( 'NONE',  ( 5.967832595844252630, 9.000000000000000000, -3.153961652902406154 ) ) ;
#2608=ORIENTED_EDGE ( 'NONE', *, *, #7398, .F. ) ;
#2616=DIRECTION ( 'NONE',  ( 0.000000000000000000, 1.000000000000000000, -0.000000000000000000 ) ) ;
#2619=EDGE_CURVE ( 'NONE', #11339, #10516, #1462, .T. ) ;
#2625=EDGE_LOOP ( 'NONE', ( #3351, #9646, #11379, #4240 ) ) ;
#2626=CARTESIAN_POINT ( 'NONE',  ( 6.736042615721505200, 9.000000000000000000, 5.184180733653466433 ) ) ;
#2656=CARTESIAN_POINT ( 'NONE',  ( 5.985774866078161338, 0.000000000000000000, 3.119775513178307147 ) ) ;
#2671=CARTESIAN_POINT ( 'NONE',  ( -6.057461899949976747, 0.000000000000000000, 5.137313564148215939 ) ) ;
#2672=CARTESIAN_POINT ( 'NONE',  ( -7.125870497355421662, 9.000000000000000000, -3.507536778237742237 ) ) ;
#2675=ORIENTED_EDGE ( 'NONE', *, *, #2310, .F. ) ;
#2678=EDGE_CURVE ( 'NONE', #4801, #9824, #12623, .T. ) ;
#2679=VECTOR ( 'NONE', #11755, 1000.000000000000000 ) ;
#2697=EDGE_CURVE ( 'NONE', #9762, #10809, #4786, .T. ) ;
#2699=DIRECTION ( 'NONE',  ( -0.000000000000000000, -1.000000000000000000, -0.000000000000000000 ) ) ;
#2703=EDGE_CURVE ( 'NONE', #933, #7402, #11531, .T. ) ;
#2715=DIRECTION ( 'NONE',  ( -0.000000000000000000, -1.000000000000000000, -0.000000000000000000 ) ) ;
#2718=ADVANCED_FACE ( 'NONE', ( #11928 ), #365, .T. ) ;
#2733=EDGE_CURVE ( 'NONE', #10192, #8876, #5097, .T. ) ;
#2737=VERTEX_POINT ( 'NONE', #12491 ) ;
#2738=ORIENTED_EDGE ( 'NONE', *, *, #2678, .F. ) ;
#2746=CIRCLE ( 'NONE', #11333, 6.750000000000000888 ) ;
#2755=VERTEX_POINT ( 'NONE', #900 ) ;
#2757=ORIENTED_EDGE ( 'NONE', *, *, #4870, .T. ) ;
#2770=ORIENTED_EDGE ( 'NONE', *, *, #8658, .T. ) ;
#2772=CARTESIAN_POINT ( 'NONE',  ( 7.151505841916629080, -1.694065894508600678E-18, 1.752496229622501511 ) ) ;
#2778=CARTESIAN_POINT ( 'NONE',  ( 0.000000000000000000, 0.000000000000000000, 0.000000000000000000 ) ) ;
#2779=CARTESIAN_POINT ( 'NONE',  ( 7.110882674384088276, 9.000000000000000000, -3.538387050178523729 ) ) ;
#2783=CARTESIAN_POINT ( 'NONE',  ( -3.833392836528145331, 1.734723475976807094E-15, -5.555861711818853799 ) ) ;
#2786=CARTESIAN_POINT ( 'NONE',  ( -7.363095878837111030, 9.000000000000000000, 0.009895496992605581216 ) ) ;
#2790=VERTEX_POINT ( 'NONE', #10330 ) ;
#2793=EDGE_CURVE ( 'NONE', #4332, #9873, #11627, .T. ) ;
#2795=DIRECTION ( 'NONE',  ( 0.000000000000000000, 1.000000000000000000, -0.000000000000000000 ) ) ;
#2798=CARTESIAN_POINT ( 'NONE',  ( 0.000000000000000000, -3.000000000000000000, 9.250000000000000000 ) ) ;
#2810=CARTESIAN_POINT ( 'NONE',  ( -0.8123631076467130452, 1.734723475976807094E-15, -6.700937709107178009 ) ) ;
#2819=ORIENTED_EDGE ( 'NONE', *, *, #12994, .T. ) ;
#2829=B_SPLINE_CURVE_WITH_KNOTS ( 'NONE', 3,
 ( #723, #7871, #4919, #2783 ),
 .UNSPECIFIED., .F., .F.,
 ( 4, 4 ),
 ( 0.1276832474596281686, 1.000000000000000000 ),
 .UNSPECIFIED. ) ;
#2830=DIRECTION ( 'NONE',  ( -0.000000000000000000, -1.000000000000000000, -0.000000000000000000 ) ) ;
#2842=DIRECTION ( 'NONE',  ( 0.000000000000000000, 1.000000000000000000, -0.000000000000000000 ) ) ;
#2854=ADVANCED_FACE ( 'NONE', ( #3860 ), #262, .T. ) ;
#2855=ORIENTED_EDGE ( 'NONE', *, *, #7920, .T. ) ;
#2862=CARTESIAN_POINT ( 'NONE',  ( 5.504794476853524188, -1.694065894508600678E-18, -4.890042597913815570 ) ) ;
#2866=ORIENTED_EDGE ( 'NONE', *, *, #2906, .T. ) ;
#2868=CARTESIAN_POINT ( 'NONE',  ( 0.000000000000000000, -3.000000000000000000, 0.000000000000000000 ) ) ;
#2878=CARTESIAN_POINT ( 'NONE',  ( 0.000000000000000000, 9.000000000000000000, 0.000000000000000000 ) ) ;
#2888=EDGE_LOOP ( 'NONE', ( #9425, #10381, #6325, #10905 ) ) ;
#2897=CARTESIAN_POINT ( 'NONE',  ( -2.590203375110137873, 0.000000000000000000, 6.893050072893555758 ) ) ;
#2899=CARTESIAN_POINT ( 'NONE',  ( 0.000000000000000000, 9.000000000000000000, 0.000000000000000000 ) ) ;
#2906=EDGE_CURVE ( 'NONE', #4948, #11926, #4310, .T. ) ;
#2917=CARTESIAN_POINT ( 'NONE',  ( 2.601737331980797041, 9.000000000000000000, -6.888123234756056590 ) ) ;
#2925=DIRECTION ( 'NONE',  ( 0.000000000000000000, 0.000000000000000000, 1.000000000000000000 ) ) ;
#2943=CARTESIAN_POINT ( 'NONE',  ( 5.051606143860416509, 9.000000000000000000, 4.477027514692274224 ) ) ;
#2944=VECTOR ( 'NONE', #11871, 1000.000000000000000 ) ;
#2948=CYLINDRICAL_SURFACE ( 'NONE', #11212, 6.750000000000001776 ) ;
#2960=CARTESIAN_POINT ( 'NONE',  ( 6.554160776451332993, 9.000000000000000000, -1.614148852004323675 ) ) ;
#2971=ADVANCED_FACE ( 'NONE', ( #8587 ), #1712, .T. ) ;
#2972=CARTESIAN_POINT ( 'NONE',  ( 0.4639228963249704130, 0.000000000000000000, 8.487330295579726069 ) ) ;
#2974=CARTESIAN_POINT ( 'NONE',  ( 1.580708947611198623, 0.000000000000000000, -8.351727918397600092 ) ) ;
#2979=CIRCLE ( 'NONE', #138, 8.499999999999998224 ) ;
#2992=CARTESIAN_POINT ( 'NONE',  ( 4.164551629694410728, 0.000000000000000000, -6.072874324029720050 ) ) ;
#2997=CARTESIAN_POINT ( 'NONE',  ( -2.481593227817846525, 9.000000000000000000, -8.129679886173168057 ) ) ;
#2999=PRODUCT_DEFINITION_FORMATION_WITH_SPECIFIED_SOURCE ( 'ANY', '', #10857, .NOT_KNOWN. ) ;
#3000=ORIENTED_EDGE ( 'NONE', *, *, #1698, .F. ) ;
#3011=DIRECTION ( 'NONE',  ( 0.000000000000000000, 0.000000000000000000, 1.000000000000000000 ) ) ;
#3014=CYLINDRICAL_SURFACE ( 'NONE', #7545, 6.750000000000000888 ) ;
#3026=EDGE_CURVE ( 'NONE', #7708, #13219, #4190, .T. ) ;
#3029=B_SPLINE_SURFACE_WITH_KNOTS ( 'NONE', 3, 1, ( 
 ( #10782, #586 ),
 ( #11761, #7937 ),
 ( #2779, #1350 ),
 ( #6986, #8644 ) ),
 .UNSPECIFIED., .F., .F., .F.,
 ( 4, 4 ),
 ( 2, 2 ),
 ( 0.000000000000000000, 0.8724294488011762327 ),
 ( 0.000000000000000000, 1.000000000000000000 ),
 .UNSPECIFIED. ) ;
#3034=CARTESIAN_POINT ( 'NONE',  ( 1.127406311874972422, 9.000000000000000000, -7.862174656777307646 ) ) ;
#3039=ORIENTED_EDGE ( 'NONE', *, *, #5146, .T. ) ;
#3040=CARTESIAN_POINT ( 'NONE',  ( 8.093005444143644311, 9.000000000000000000, -2.598704077239528232 ) ) ;
#3052=DIRECTION ( 'NONE',  ( -0.000000000000000000, 1.000000000000000000, -0.000000000000000000 ) ) ;
#3073=EDGE_LOOP ( 'NONE', ( #8720, #10119, #5212, #1076 ) ) ;
#3074=CARTESIAN_POINT ( 'NONE',  ( -7.155006492985575228, 0.000000000000000000, -1.740452503570284915 ) ) ;
#3075=CIRCLE ( 'NONE', #5088, 8.499999999999992895 ) ;
#3080=CARTESIAN_POINT ( 'NONE',  ( 0.000000000000000000, 0.000000000000000000, 0.000000000000000000 ) ) ;
#3100=CARTESIAN_POINT ( 'NONE',  ( -2.632142621505047408, 0.000000000000000000, -6.877144614729746586 ) ) ;
#3106=DIRECTION ( 'NONE',  ( 0.000000000000000000, 0.000000000000000000, 1.000000000000000000 ) ) ;
#3124=VERTEX_POINT ( 'NONE', #1444 ) ;
#3130=VECTOR ( 'NONE', #2699, 1000.000000000000000 ) ;
#3135=ADVANCED_FACE ( 'NONE', ( #7771 ), #5634, .T. ) ;
#3142=AXIS2_PLACEMENT_3D ( 'NONE', #11090, #5854, #1514 ) ;
#3150=B_SPLINE_CURVE_WITH_KNOTS ( 'NONE', 3,
 ( #12535, #3074, #7288, #6888 ),
 .UNSPECIFIED., .F., .F.,
 ( 4, 4 ),
 ( 0.000000000000000000, 0.8724294488011763438 ),
 .UNSPECIFIED. ) ;
#3165=EDGE_CURVE ( 'NONE', #8551, #8134, #3635, .T. ) ;
#3175=ORIENTED_EDGE ( 'NONE', *, *, #11211, .T. ) ;
#3182=EDGE_CURVE ( 'NONE', #10584, #479, #5564, .T. ) ;
#3187=CARTESIAN_POINT ( 'NONE',  ( -2.655466033450426533, 0.000000000000000000, -7.485541762018160128 ) ) ;
#3189=CARTESIAN_POINT ( 'NONE',  ( -5.976238463952679325, 0.000000000000000000, -3.138004751744733589 ) ) ;
#3192=DIRECTION ( 'NONE',  ( -0.000000000000000000, -1.000000000000000000, -0.000000000000000000 ) ) ;
#3196=VERTEX_POINT ( 'NONE', #5013 ) ;
#3209=ORIENTED_EDGE ( 'NONE', *, *, #9198, .T. ) ;
#3214=CARTESIAN_POINT ( 'NONE',  ( 2.458659560121116527, 9.000000000000000000, -8.136645080586040635 ) ) ;
#3221=CARTESIAN_POINT ( 'NONE',  ( 3.850308450823737516, 9.000000000000000000, 5.544152309732777617 ) ) ;
#3235=B_SPLINE_CURVE_WITH_KNOTS ( 'NONE', 3,
 ( #5395, #2499, #3252, #4425 ),
 .UNSPECIFIED., .F., .F.,
 ( 4, 4 ),
 ( 0.1276832474596238665, 1.000000000000000000 ),
 .UNSPECIFIED. ) ;
#3237=CARTESIAN_POINT ( 'NONE',  ( 6.749972395921142621, 9.000000000000000000, -0.01930425607464712062 ) ) ;
#3250=CARTESIAN_POINT ( 'NONE',  ( 5.517918333394296049, -1.694065894508600678E-18, 4.875228826198821253 ) ) ;
#3252=CARTESIAN_POINT ( 'NONE',  ( 2.620242232815953809, 9.000000000000000000, 6.881105251569436199 ) ) ;
#3254=VERTEX_POINT ( 'NONE', #1782 ) ;
#3263=EDGE_CURVE ( 'NONE', #9464, #1815, #12097, .T. ) ;
#3269=PLANE ( 'NONE',  #2214 ) ;
#3273=DIRECTION ( 'NONE',  ( 0.000000000000000000, 1.000000000000000000, -0.000000000000000000 ) ) ;
#3274=EDGE_CURVE ( 'NONE', #12645, #3761, #7687, .T. ) ;
#3285=ORIENTED_EDGE ( 'NONE', *, *, #5922, .F. ) ;
#3290=CARTESIAN_POINT ( 'NONE',  ( -6.558450276537426404, 9.000000000000000000, -1.596630818375420757 ) ) ;
#3297=CARTESIAN_POINT ( 'NONE',  ( 3.818534268238711782, 9.000000000000000000, -5.566084444408534004 ) ) ;
#3299=ADVANCED_FACE ( 'NONE', ( #8173 ), #2948, .T. ) ;
#3302=DIRECTION ( 'NONE',  ( 0.000000000000000000, 1.000000000000000000, -0.000000000000000000 ) ) ;
#3309=B_SPLINE_CURVE_WITH_KNOTS ( 'NONE', 3,
 ( #6356, #8287, #3250, #2096 ),
 .UNSPECIFIED., .F., .F.,
 ( 4, 4 ),
 ( 0.1276832474596250877, 1.000000000000000000 ),
 .UNSPECIFIED. ) ;
#3322=B_SPLINE_CURVE_WITH_KNOTS ( 'NONE', 3,
 ( #9469, #126, #10371, #12528 ),
 .UNSPECIFIED., .F., .F.,
 ( 4, 4 ),
 ( 0.1276832474596231171, 1.000000000000000000 ),
 .UNSPECIFIED. ) ;
#3326=CARTESIAN_POINT ( 'NONE',  ( 2.623034112301249721, -1.694065894508600678E-18, -7.496701717520498853 ) ) ;
#3328=CARTESIAN_POINT ( 'NONE',  ( 7.363612555047485131, 9.000000000000000000, -0.02242701489043354146 ) ) ;
#3340=B_SPLINE_CURVE_WITH_KNOTS ( 'NONE', 3,
 ( #6905, #1889, #7191, #4980 ),
 .UNSPECIFIED., .F., .F.,
 ( 4, 4 ),
 ( 0.1276832474596244493, 1.000000000000000000 ),
 .UNSPECIFIED. ) ;
#3342=FACE_OUTER_BOUND ( 'NONE', #5858, .T. ) ;
#3343=CIRCLE ( 'NONE', #1152, 8.499999999999998224 ) ;
#3345=AXIS2_PLACEMENT_3D ( 'NONE', #11461, #2030, #2161 ) ;
#3351=ORIENTED_EDGE ( 'NONE', *, *, #5080, .T. ) ;
#3354=ORIENTED_EDGE ( 'NONE', *, *, #4091, .F. ) ;
#3364=FACE_OUTER_BOUND ( 'NONE', #266, .T. ) ;
#3368=CARTESIAN_POINT ( 'NONE',  ( -8.479748006907131597, 9.000000000000000000, 0.5864074857593127854 ) ) ;
#3376=EDGE_LOOP ( 'NONE', ( #3723, #6204, #237, #4823 ) ) ;
#3381=DIRECTION ( 'NONE',  ( 0.000000000000000000, 0.000000000000000000, 1.000000000000000000 ) ) ;
#3389=B_SPLINE_SURFACE_WITH_KNOTS ( 'NONE', 3, 1, ( 
 ( #12837, #6354 ),
 ( #10759, #4359 ),
 ( #11863, #1397 ),
 ( #9793, #8747 ) ),
 .UNSPECIFIED., .F., .F., .F.,
 ( 4, 4 ),
 ( 2, 2 ),
 ( 0.1276832474596256706, 1.000000000000000000 ),
 ( 0.000000000000000000, 1.000000000000000000 ),
 .UNSPECIFIED. ) ;
#3390=CARTESIAN_POINT ( 'NONE',  ( -3.835481108877868195, 9.000000000000000000, 5.554420281491219136 ) ) ;
#3395=CIRCLE ( 'NONE', #9988, 0.4000000000000000222 ) ;
#3397=EDGE_LOOP ( 'NONE', ( #12820, #7449, #235, #10058 ) ) ;
#3404=LINE ( 'NONE', #11877, #10147 ) ;
#3411=EDGE_CURVE ( 'NONE', #2737, #3746, #1022, .T. ) ;
#3420=EDGE_LOOP ( 'NONE', ( #9911, #1329 ) ) ;
#3426=ORIENTED_EDGE ( 'NONE', *, *, #11384, .T. ) ;
#3432=CARTESIAN_POINT ( 'NONE',  ( -5.496871281090180972, 9.000000000000000000, 4.899765193453235135 ) ) ;
#3443=B_SPLINE_SURFACE_WITH_KNOTS ( 'NONE', 3, 1, ( 
 ( #3290, #12746 ),
 ( #5497, #155 ),
 ( #9577, #8285 ),
 ( #5370, #1959 ) ),
 .UNSPECIFIED., .F., .F., .F.,
 ( 4, 4 ),
 ( 2, 2 ),
 ( 0.000000000000000000, 0.8724294488011763438 ),
 ( 0.000000000000000000, 1.000000000000000000 ),
 .UNSPECIFIED. ) ;
#3446=( NAMED_UNIT ( * ) SI_UNIT ( $, .STERADIAN. ) SOLID_ANGLE_UNIT ( ) );
#3454=B_SPLINE_SURFACE_WITH_KNOTS ( 'NONE', 3, 1, ( 
 ( #3464, #5606 ),
 ( #3328, #439 ),
 ( #9808, #10771 ),
 ( #1413, #2373 ) ),
 .UNSPECIFIED., .F., .F., .F.,
 ( 4, 4 ),
 ( 2, 2 ),
 ( 0.000000000000000000, 0.8724294488011776760 ),
 ( 0.000000000000000000, 1.000000000000000000 ),
 .UNSPECIFIED. ) ;
#3464=CARTESIAN_POINT ( 'NONE',  ( 6.749972395921142621, 9.000000000000000000, -0.01930425607464666612 ) ) ;
#3471=CARTESIAN_POINT ( 'NONE',  ( 4.369710415961185035, 0.000000000000000000, 6.632530905044255576 ) ) ;
#3485=CARTESIAN_POINT ( 'NONE',  ( 0.000000000000000000, 9.000000000000000000, 0.000000000000000000 ) ) ;
#3487=ORIENTED_EDGE ( 'NONE', *, *, #6250, .F. ) ;
#3489=EDGE_LOOP ( 'NONE', ( #7681, #1050, #2384, #10735 ) ) ;
#3498=VERTEX_POINT ( 'NONE', #11043 ) ;
#3503=VERTEX_POINT ( 'NONE', #9751 ) ;
#3505=EDGE_LOOP ( 'NONE', ( #9109, #10052, #8894, #3426 ) ) ;
#3517=ORIENTED_EDGE ( 'NONE', *, *, #13257, .T. ) ;
#3519=ORIENTED_EDGE ( 'NONE', *, *, #7769, .T. ) ;
#3522=VECTOR ( 'NONE', #13167, 1000.000000000000000 ) ;
#3529=ADVANCED_FACE ( 'NONE', ( #7557 ), #11827, .T. ) ;
#3530=DIRECTION ( 'NONE',  ( 0.000000000000000000, 0.000000000000000000, 1.000000000000000000 ) ) ;
#3531=AXIS2_PLACEMENT_3D ( 'NONE', #12529, #10372, #941 ) ;
#3535=CARTESIAN_POINT ( 'NONE',  ( -2.375523406013128280, 0.000000000000000000, 6.318179211409232998 ) ) ;
#3536=ADVANCED_FACE ( 'NONE', ( #3342 ), #3029, .T. ) ;
#3562=CIRCLE ( 'NONE', #7962, 9.250000000000000000 ) ;
#3577=LINE ( 'NONE', #4549, #1819 ) ;
#3581=EDGE_CURVE ( 'NONE', #5694, #7353, #11439, .T. ) ;
#3583=CIRCLE ( 'NONE', #9091, 6.750000000000001776 ) ;
#3588=CARTESIAN_POINT ( 'NONE',  ( 0.000000000000000000, 9.000000000000000000, 0.000000000000000000 ) ) ;
#3599=CARTESIAN_POINT ( 'NONE',  ( -6.749999880766614169, 1.734723475976807094E-15, -0.001268720102703522860 ) ) ;
#3606=CARTESIAN_POINT ( 'NONE',  ( -7.939678587550617728, 0.000000000000000000, 0.2057875656132798770 ) ) ;
#3610=DIRECTION ( 'NONE',  ( 0.000000000000000000, 0.000000000000000000, -1.000000000000000000 ) ) ;
#3620=DIRECTION ( 'NONE',  ( -0.000000000000000000, -1.000000000000000000, -0.000000000000000000 ) ) ;
#3623=DIRECTION ( 'NONE',  ( -0.000000000000000000, -1.000000000000000000, -0.000000000000000000 ) ) ;
#3624=CARTESIAN_POINT ( 'NONE',  ( -7.235926821844430812, 9.000000000000000000, 4.459973433655439301 ) ) ;
#3625=DIRECTION ( 'NONE',  ( -0.000000000000000000, -1.000000000000000000, -0.000000000000000000 ) ) ;
#3635=LINE ( 'NONE', #347, #657 ) ;
#3636=DIRECTION ( 'NONE',  ( -0.000000000000000000, -1.000000000000000000, -0.000000000000000000 ) ) ;
#3638=CARTESIAN_POINT ( 'NONE',  ( 6.509732753943064054, 0.000000000000000000, -3.441899519755141412 ) ) ;
#3640=CARTESIAN_POINT ( 'NONE',  ( -1.604252589105052307, 9.000000000000000000, -8.347237484961700815 ) ) ;
#3642=FACE_OUTER_BOUND ( 'NONE', #3489, .T. ) ;
#3650=CARTESIAN_POINT ( 'NONE',  ( 0.000000000000000000, 0.000000000000000000, 0.000000000000000000 ) ) ;
#3652=CARTESIAN_POINT ( 'NONE',  ( -5.065227977808753224, 0.000000000000000000, -4.461610195077944319 ) ) ;
#3653=DIRECTION ( 'NONE',  ( 0.000000000000000000, 0.000000000000000000, 1.000000000000000000 ) ) ;
#3658=ORIENTED_EDGE ( 'NONE', *, *, #1478, .T. ) ;
#3667=CARTESIAN_POINT ( 'NONE',  ( -4.679611352264966051, 9.000000000000000000, -6.417326716594978997 ) ) ;
#3669=CARTESIAN_POINT ( 'NONE',  ( 7.248474140376191421, 0.000000000000000000, 4.439552076088042476 ) ) ;
#3675=ORIENTED_EDGE ( 'NONE', *, *, #2678, .T. ) ;
#3678=DIRECTION ( 'NONE',  ( 0.000000000000000000, 0.000000000000000000, 1.000000000000000000 ) ) ;
#3684=LINE ( 'NONE', #1494, #7574 ) ;
#3687=ORIENTED_EDGE ( 'NONE', *, *, #11709, .T. ) ;
#3695=CARTESIAN_POINT ( 'NONE',  ( 6.554160776451332104, 9.000000000000000000, -1.614148852004323231 ) ) ;
#3696=CARTESIAN_POINT ( 'NONE',  ( 5.958322434183388694, 0.000000000000000000, -6.062045345451230638 ) ) ;
#3718=CARTESIAN_POINT ( 'NONE',  ( -5.065227977808755000, 0.000000000000000000, -4.461610195077942542 ) ) ;
#3721=DIRECTION ( 'NONE',  ( -0.000000000000000000, -1.000000000000000000, -0.000000000000000000 ) ) ;
#3723=ORIENTED_EDGE ( 'NONE', *, *, #2906, .F. ) ;
#3732=DIRECTION ( 'NONE',  ( -0.000000000000000000, -1.000000000000000000, -0.000000000000000000 ) ) ;
#3742=VERTEX_POINT ( 'NONE', #7395 ) ;
#3743=ORIENTED_EDGE ( 'NONE', *, *, #9108, .T. ) ;
#3746=VERTEX_POINT ( 'NONE', #1192 ) ;
#3751=AXIS2_PLACEMENT_3D ( 'NONE', #11289, #5909, #8250 ) ;
#3752=EDGE_CURVE ( 'NONE', #4948, #175, #6417, .T. ) ;
#3761=VERTEX_POINT ( 'NONE', #11730 ) ;
#3764=CYLINDRICAL_SURFACE ( 'NONE', #11061, 8.500000000000000000 ) ;
#3771=CARTESIAN_POINT ( 'NONE',  ( -6.524296280129988190, 9.000000000000000000, -3.413039245436654490 ) ) ;
#3773=CARTESIAN_POINT ( 'NONE',  ( -1.161309641800940540, 9.000000000000000000, -7.856984441350959969 ) ) ;
#3795=EDGE_LOOP ( 'NONE', ( #2500, #8434, #8534, #11867 ) ) ;
#3800=CARTESIAN_POINT ( 'NONE',  ( 6.749972395921142621, 9.000000000000000000, -0.01930425607464712062 ) ) ;
#3806=CARTESIAN_POINT ( 'NONE',  ( -7.363095878837111030, -1.694065894508600678E-18, 0.009895496992605581216 ) ) ;
#3823=EDGE_LOOP ( 'NONE', ( #4203, #3743, #2866, #1068, #2770, #7948, #12136, #9629, #9158, #8873, #8668, #4928, #5204, #2273, #9207, #4995, #564, #4909, #11246, #5690, #2819, #6689, #10302, #9159, #2048, #10641, #1324, #12710, #2757, #9330, #6734, #4744, #7015, #6628, #1485, #4025, #5914, #12033, #5957, #400, #1292, #5107, #4531, #5439, #8975, #3487, #1906, #5185, #1516, #7534, #11837, #12520, #754 ) ) ;
#3837=CIRCLE ( 'NONE', #11097, 8.499999999999998224 ) ;
#3841=ORIENTED_EDGE ( 'NONE', *, *, #4998, .T. ) ;
#3842=DIRECTION ( 'NONE',  ( 0.000000000000000000, 0.000000000000000000, 1.000000000000000000 ) ) ;
#3860=FACE_OUTER_BOUND ( 'NONE', #363, .T. ) ;
#3868=ORIENTED_EDGE ( 'NONE', *, *, #9266, .T. ) ;
#3870=VERTEX_POINT ( 'NONE', #1255 ) ;
#3872=LINE ( 'NONE', #8077, #3130 ) ;
#3881=LINE ( 'NONE', #10979, #13456 ) ;
#3883=CARTESIAN_POINT ( 'NONE',  ( 3.818534268238711782, 9.000000000000000000, -5.566084444408534004 ) ) ;
#3888=ORIENTED_EDGE ( 'NONE', *, *, #11545, .F. ) ;
#3908=CARTESIAN_POINT ( 'NONE',  ( -5.976238463952679325, 9.000000000000000000, -3.138004751744734477 ) ) ;
#3918=VERTEX_POINT ( 'NONE', #12072 ) ;
#3923=CARTESIAN_POINT ( 'NONE',  ( 3.007863545083557355, 9.000000000000000000, 7.350755164602351677 ) ) ;
#3924=CARTESIAN_POINT ( 'NONE',  ( -5.299649803506881085, 0.000000000000000000, -6.645578376649351249 ) ) ;
#3927=CARTESIAN_POINT ( 'NONE',  ( 0.000000000000000000, 9.000000000000000000, 0.000000000000000000 ) ) ;
#3929=EDGE_LOOP ( 'NONE', ( #1047, #5271, #10475, #4064 ) ) ;
#3930=CARTESIAN_POINT ( 'NONE',  ( -2.655466033450426533, 0.000000000000000000, -7.485541762018160128 ) ) ;
#3951=ORIENTED_EDGE ( 'NONE', *, *, #141, .F. ) ;
#3952=EDGE_CURVE ( 'NONE', #10761, #10809, #8331, .T. ) ;
#3953=EDGE_CURVE ( 'NONE', #76, #11033, #10959, .T. ) ;
#3954=ORIENTED_EDGE ( 'NONE', *, *, #3274, .F. ) ;
#3967=DIRECTION ( 'NONE',  ( 0.000000000000000000, 1.000000000000000000, -0.000000000000000000 ) ) ;
#3978=CARTESIAN_POINT ( 'NONE',  ( -5.039625798601655937, 9.000000000000000000, 4.490509081392511703 ) ) ;
#3989=ADVANCED_FACE ( 'NONE', ( #11931 ), #13558, .T. ) ;
#4003=ORIENTED_EDGE ( 'NONE', *, *, #3953, .T. ) ;
#4004=CARTESIAN_POINT ( 'NONE',  ( -2.481593227817846525, 9.000000000000000000, -8.129679886173168057 ) ) ;
#4006=ADVANCED_FACE ( 'NONE', ( #12430 ), #10128, .T. ) ;
#4009=B_SPLINE_CURVE_WITH_KNOTS ( 'NONE', 3,
 ( #3040, #10554, #11652, #7251 ),
 .UNSPECIFIED., .F., .F.,
 ( 4, 4 ),
 ( 0.1276832474596231171, 1.000000000000000000 ),
 .UNSPECIFIED. ) ;
#4018=CARTESIAN_POINT ( 'NONE',  ( -7.780961115628988622, 0.000000000000000000, -3.421497350147985728 ) ) ;
#4019=B_SPLINE_SURFACE_WITH_KNOTS ( 'NONE', 3, 1, ( 
 ( #8729, #8862 ),
 ( #11844, #2403 ),
 ( #4808, #8935 ),
 ( #3695, #7897 ) ),
 .UNSPECIFIED., .F., .F., .F.,
 ( 4, 4 ),
 ( 2, 2 ),
 ( 0.1276832474596231171, 1.000000000000000000 ),
 ( 0.000000000000000000, 1.000000000000000000 ),
 .UNSPECIFIED. ) ;
#4025=ORIENTED_EDGE ( 'NONE', *, *, #8257, .F. ) ;
#4026=AXIS2_PLACEMENT_3D ( 'NONE', #8261, #12739, #12880 ) ;
#4031=CARTESIAN_POINT ( 'NONE',  ( -7.780961115628980629, 0.000000000000000000, -3.421497350147988392 ) ) ;
#4034=CARTESIAN_POINT ( 'NONE',  ( -5.039625798601655937, 9.000000000000000000, 4.490509081392509927 ) ) ;
#4043=CARTESIAN_POINT ( 'NONE',  ( 7.940744365623959133, 0.000000000000000000, 0.1715058177969961128 ) ) ;
#4046=EDGE_LOOP ( 'NONE', ( #10240, #6959, #10748, #4615 ) ) ;
#4051=AXIS2_PLACEMENT_3D ( 'NONE', #12470, #7216, #6172 ) ;
#4054=ADVANCED_FACE ( 'NONE', ( #10332 ), #12399, .T. ) ;
#4055=CARTESIAN_POINT ( 'NONE',  ( -7.125870497355421662, 0.000000000000000000, -3.507536778237742237 ) ) ;
#4064=ORIENTED_EDGE ( 'NONE', *, *, #2232, .T. ) ;
#4067=CIRCLE ( 'NONE', #13539, 0.4000000000000000222 ) ;
#4068=CARTESIAN_POINT ( 'NONE',  ( 2.620242232815953809, 0.000000000000000000, 6.881105251569436199 ) ) ;
#4071=DIRECTION ( 'NONE',  ( 0.000000000000000000, 1.000000000000000000, -0.000000000000000000 ) ) ;
#4075=ORIENTED_EDGE ( 'NONE', *, *, #10649, .T. ) ;
#4078=AXIS2_PLACEMENT_3D ( 'NONE', #8717, #3273, #2186 ) ;
#4091=EDGE_CURVE ( 'NONE', #7238, #3870, #4851, .T. ) ;
#4095=ORIENTED_EDGE ( 'NONE', *, *, #11148, .T. ) ;
#4101=ORIENTED_EDGE ( 'NONE', *, *, #6279, .T. ) ;
#4124=EDGE_LOOP ( 'NONE', ( #658, #3000, #7192, #2586 ) ) ;
#4127=B_SPLINE_CURVE_WITH_KNOTS ( 'NONE', 3,
 ( #9355, #8443, #4174, #1079 ),
 .UNSPECIFIED., .F., .F.,
 ( 4, 4 ),
 ( 0.1276832474596281686, 1.000000000000000000 ),
 .UNSPECIFIED. ) ;
#4132=CARTESIAN_POINT ( 'NONE',  ( 0.7868956173019259204, 9.000000000000000000, 7.903520140620750034 ) ) ;
#4134=EDGE_CURVE ( 'NONE', #1296, #672, #4631, .T. ) ;
#4135=CARTESIAN_POINT ( 'NONE',  ( 0.8653219153705552502, 0.000000000000000000, -7.312626806738413698 ) ) ;
#4137=ORIENTED_EDGE ( 'NONE', *, *, #11384, .F. ) ;
#4145=CYLINDRICAL_SURFACE ( 'NONE', #10002, 6.749999999999999112 ) ;
#4147=CARTESIAN_POINT ( 'NONE',  ( 5.280889752749253319, 9.000000000000000000, -6.660495733750448011 ) ) ;
#4150=CARTESIAN_POINT ( 'NONE',  ( -6.549210654805285081, 9.000000000000000000, 1.634117437329677180 ) ) ;
#4151=ADVANCED_FACE ( 'NONE', ( #10609 ), #2195, .T. ) ;
#4152=CARTESIAN_POINT ( 'NONE',  ( -4.340891659662447388, 0.000000000000000000, 6.651128039276029469 ) ) ;
#4153=CARTESIAN_POINT ( 'NONE',  ( -5.976238463952679325, 0.000000000000000000, -3.138004751744733589 ) ) ;
#4174=CARTESIAN_POINT ( 'NONE',  ( -4.190859029938718727, 9.000000000000000000, -6.054087828318142073 ) ) ;
#4181=CARTESIAN_POINT ( 'NONE',  ( 4.898587196589413075E-17, 9.000000000000000000, 0.4000000000000000222 ) ) ;
#4190=LINE ( 'NONE', #5229, #221 ) ;
#4197=DIRECTION ( 'NONE',  ( 0.000000000000000000, 0.000000000000000000, -1.000000000000000000 ) ) ;
#4199=ORIENTED_EDGE ( 'NONE', *, *, #3274, .T. ) ;
#4200=CARTESIAN_POINT ( 'NONE',  ( -2.411622991978543684, 0.000000000000000000, -6.304488444319686913 ) ) ;
#4203=ORIENTED_EDGE ( 'NONE', *, *, #2703, .F. ) ;
#4209=CARTESIAN_POINT ( 'NONE',  ( 2.601737331980797041, 0.000000000000000000, -6.888123234756056590 ) ) ;
#4211=CARTESIAN_POINT ( 'NONE',  ( -2.411622991978541464, 0.000000000000000000, -6.304488444319688689 ) ) ;
#4218=FACE_OUTER_BOUND ( 'NONE', #3823, .T. ) ;
#4225=ADVANCED_FACE ( 'NONE', ( #12052 ), #4019, .T. ) ;
#4239=ORIENTED_EDGE ( 'NONE', *, *, #10280, .T. ) ;
#4240=ORIENTED_EDGE ( 'NONE', *, *, #290, .T. ) ;
#4243=ORIENTED_EDGE ( 'NONE', *, *, #11709, .F. ) ;
#4247=AXIS2_PLACEMENT_3D ( 'NONE', #8626, #2436, #3530 ) ;
#4252=LINE ( 'NONE', #4527, #12440 ) ;
#4259=ORIENTED_EDGE ( 'NONE', *, *, #10875, .T. ) ;
#4262=CARTESIAN_POINT ( 'NONE',  ( 0.7944557581062196006, 9.000000000000000000, -6.703084368289862205 ) ) ;
#4270=CIRCLE ( 'NONE', #6043, 6.750000000000000888 ) ;
#4271=CARTESIAN_POINT ( 'NONE',  ( 0.000000000000000000, 0.000000000000000000, 0.000000000000000000 ) ) ;
#4287=EDGE_CURVE ( 'NONE', #5612, #10060, #7071, .T. ) ;
#4292=VECTOR ( 'NONE', #3192, 1000.000000000000000 ) ;
#4304=CARTESIAN_POINT ( 'NONE',  ( 4.355042381134428098, 0.000000000000000000, 7.299562031966232212 ) ) ;
#4310=CIRCLE ( 'NONE', #2272, 6.750000000000000888 ) ;
#4315=ADVANCED_FACE ( 'NONE', ( #405 ), #11007, .T. ) ;
#4316=EDGE_LOOP ( 'NONE', ( #10818, #8516, #12803, #10935 ) ) ;
#4319=ORIENTED_EDGE ( 'NONE', *, *, #13491, .T. ) ;
#4327=EDGE_CURVE ( 'NONE', #2790, #8976, #4676, .T. ) ;
#4332=VERTEX_POINT ( 'NONE', #4540 ) ;
#4338=CARTESIAN_POINT ( 'NONE',  ( -5.977417671213807182, 0.000000000000000000, 3.135757960025121527 ) ) ;
#4341=CARTESIAN_POINT ( 'NONE',  ( 0.000000000000000000, -3.000000000000000000, 0.000000000000000000 ) ) ;
#4359=CARTESIAN_POINT ( 'NONE',  ( -0.7527353566742582824, 0.000000000000000000, 7.906594341344654886 ) ) ;
#4360=CARTESIAN_POINT ( 'NONE',  ( -3.835481108877868195, 9.000000000000000000, 5.554420281491219136 ) ) ;
#4370=CARTESIAN_POINT ( 'NONE',  ( 0.000000000000000000, 9.000000000000000000, -6.750000000000000888 ) ) ;
#4379=VERTEX_POINT ( 'NONE', #9361 ) ;
#4386=LINE ( 'NONE', #1287, #6039 ) ;
#4418=CARTESIAN_POINT ( 'NONE',  ( -0.8123631076467130452, 9.000000000000000000, -6.700937709107179785 ) ) ;
#4419=CARTESIAN_POINT ( 'NONE',  ( 0.000000000000000000, 9.000000000000000000, -6.750000000000000888 ) ) ;
#4425=CARTESIAN_POINT ( 'NONE',  ( 2.392396671352952087, 9.000000000000000000, 6.311809420990097230 ) ) ;
#4428=VECTOR ( 'NONE', #9936, 1000.000000000000000 ) ;
#4432=EDGE_LOOP ( 'NONE', ( #5325, #3888, #2128, #4075 ) ) ;
#4436=CARTESIAN_POINT ( 'NONE',  ( -8.369528376005813897, 9.000000000000000000, 1.483574994138652903 ) ) ;
#4441=AXIS2_PLACEMENT_3D ( 'NONE', #2868, #13555, #8367 ) ;
#4447=DIRECTION ( 'NONE',  ( 0.000000000000000000, 0.000000000000000000, -1.000000000000000000 ) ) ;
#4450=DIRECTION ( 'NONE',  ( 0.000000000000000000, -1.000000000000000000, 0.000000000000000000 ) ) ;
#4467=EDGE_CURVE ( 'NONE', #11339, #2737, #12125, .T. ) ;
#4470=EDGE_CURVE ( 'NONE', #12047, #1815, #10105, .T. ) ;
#4471=AXIS2_PLACEMENT_3D ( 'NONE', #2243, #12665, #6452 ) ;
#4472=DIRECTION ( 'NONE',  ( 0.000000000000000000, -1.000000000000000000, 0.000000000000000000 ) ) ;
#4486=ORIENTED_EDGE ( 'NONE', *, *, #5965, .F. ) ;
#4489=CIRCLE ( 'NONE', #13075, 8.499999999999998224 ) ;
#4499=FACE_OUTER_BOUND ( 'NONE', #3929, .T. ) ;
#4502=EDGE_LOOP ( 'NONE', ( #6162, #6163, #11562, #1182 ) ) ;
#4515=ORIENTED_EDGE ( 'NONE', *, *, #613, .T. ) ;
#4526=CARTESIAN_POINT ( 'NONE',  ( 6.553553527263006551, 9.000000000000000000, 1.616612558808879774 ) ) ;
#4527=CARTESIAN_POINT ( 'NONE',  ( -5.299649803506881085, 9.000000000000000000, -6.645578376649351249 ) ) ;
#4528=CARTESIAN_POINT ( 'NONE',  ( 8.093005444143644311, 0.000000000000000000, -2.598704077239528232 ) ) ;
#4529=DIRECTION ( 'NONE',  ( -0.000000000000000000, -1.000000000000000000, -0.000000000000000000 ) ) ;
#4531=ORIENTED_EDGE ( 'NONE', *, *, #9798, .T. ) ;
#4537=ORIENTED_EDGE ( 'NONE', *, *, #1057, .T. ) ;
#4538=CARTESIAN_POINT ( 'NONE',  ( -6.549210654805285081, 9.000000000000000000, 1.634117437329677180 ) ) ;
#4540=CARTESIAN_POINT ( 'NONE',  ( 6.749972395921142621, 0.000000000000000000, -0.01930425607464712062 ) ) ;
#4541=LINE ( 'NONE', #6679, #318 ) ;
#4544=ORIENTED_EDGE ( 'NONE', *, *, #2196, .T. ) ;
#4549=CARTESIAN_POINT ( 'NONE',  ( -1.604252589105048976, 9.000000000000000000, -8.347237484961699039 ) ) ;
#4551=ADVANCED_FACE ( 'NONE', ( #9483, #1024 ), #3269, .F. ) ;
#4554=DIRECTION ( 'NONE',  ( -0.000000000000000000, -1.000000000000000000, -0.000000000000000000 ) ) ;
#4564=CARTESIAN_POINT ( 'NONE',  ( 5.504794476853524188, 0.000000000000000000, -4.890042597913815570 ) ) ;
#4594=ORIENTED_EDGE ( 'NONE', *, *, #12810, .F. ) ;
#4597=EDGE_CURVE ( 'NONE', #8655, #9873, #12670, .T. ) ;
#4600=CARTESIAN_POINT ( 'NONE',  ( 5.985774866078160450, 0.000000000000000000, 3.119775513178307147 ) ) ;
#4613=DIRECTION ( 'NONE',  ( -0.000000000000000000, -1.000000000000000000, -0.000000000000000000 ) ) ;
#4615=ORIENTED_EDGE ( 'NONE', *, *, #11492, .T. ) ;
#4622=CARTESIAN_POINT ( 'NONE',  ( -5.065227977808755000, 9.000000000000000000, -4.461610195077942542 ) ) ;
#4628=ORIENTED_EDGE ( 'NONE', *, *, #1057, .F. ) ;
#4629=ORIENTED_EDGE ( 'NONE', *, *, #5312, .F. ) ;
#4631=CIRCLE ( 'NONE', #27, 9.250000000000000000 ) ;
#4635=DIRECTION ( 'NONE',  ( 0.000000000000000000, 1.000000000000000000, -0.000000000000000000 ) ) ;
#4639=ADVANCED_FACE ( 'NONE', ( #6379 ), #10591, .T. ) ;
#4643=ADVANCED_FACE ( 'NONE', ( #10786 ), #9527, .T. ) ;
#4653=CARTESIAN_POINT ( 'NONE',  ( 0.000000000000000000, 9.000000000000000000, 0.000000000000000000 ) ) ;
#4654=EDGE_CURVE ( 'NONE', #11220, #1159, #8844, .T. ) ;
#4669=ORIENTED_EDGE ( 'NONE', *, *, #9184, .T. ) ;
#4671=AXIS2_PLACEMENT_3D ( 'NONE', #8011, #13332, #10077 ) ;
#4673=DIRECTION ( 'NONE',  ( -0.000000000000000000, -1.000000000000000000, -0.000000000000000000 ) ) ;
#4674=B_SPLINE_SURFACE_WITH_KNOTS ( 'NONE', 3, 1, ( 
 ( #7688, #2656 ),
 ( #1708, #6659 ),
 ( #2528, #5754 ),
 ( #667, #4861 ) ),
 .UNSPECIFIED., .F., .F., .F.,
 ( 4, 4 ),
 ( 2, 2 ),
 ( 0.000000000000000000, 0.8724294488011774540 ),
 ( 0.000000000000000000, 1.000000000000000000 ),
 .UNSPECIFIED. ) ;
#4676=LINE ( 'NONE', #5565, #9252 ) ;
#4682=ORIENTED_EDGE ( 'NONE', *, *, #12673, .T. ) ;
#4686=VERTEX_POINT ( 'NONE', #1639 ) ;
#4690=DIRECTION ( 'NONE',  ( 0.000000000000000000, -1.000000000000000000, 0.000000000000000000 ) ) ;
#4693=AXIS2_PLACEMENT_3D ( 'NONE', #338, #4529, #10672 ) ;
#4696=CARTESIAN_POINT ( 'NONE',  ( -5.975392301194336397, 0.000000000000000000, -6.045220165289885372 ) ) ;
#4702=ORIENTED_EDGE ( 'NONE', *, *, #9188, .T. ) ;
#4710=DIRECTION ( 'NONE',  ( 0.000000000000000000, 0.000000000000000000, 1.000000000000000000 ) ) ;
#4721=ORIENTED_EDGE ( 'NONE', *, *, #6581, .F. ) ;
#4729=ADVANCED_FACE ( 'NONE', ( #13066 ), #8646, .F. ) ;
#4733=CARTESIAN_POINT ( 'NONE',  ( 5.958322434183388694, 9.000000000000000000, -6.062045345451230638 ) ) ;
#4737=DIRECTION ( 'NONE',  ( -0.000000000000000000, -1.000000000000000000, -0.000000000000000000 ) ) ;
#4744=ORIENTED_EDGE ( 'NONE', *, *, #8055, .F. ) ;
#4748=EDGE_CURVE ( 'NONE', #11943, #5243, #9050, .T. ) ;
#4750=FACE_OUTER_BOUND ( 'NONE', #46, .T. ) ;
#4753=CYLINDRICAL_SURFACE ( 'NONE', #11116, 6.749999999999999112 ) ;
#4769=CYLINDRICAL_SURFACE ( 'NONE', #5150, 6.750000000000000888 ) ;
#4773=LINE ( 'NONE', #8957, #4900 ) ;
#4777=ORIENTED_EDGE ( 'NONE', *, *, #11140, .T. ) ;
#4786=CIRCLE ( 'NONE', #12285, 8.499999999999996447 ) ;
#4801=VERTEX_POINT ( 'NONE', #7150 ) ;
#4808=CARTESIAN_POINT ( 'NONE',  ( 7.146769547044127258, 9.000000000000000000, -1.771712133291270863 ) ) ;
#4809=CARTESIAN_POINT ( 'NONE',  ( -1.161309641800940540, -1.694065894508600678E-18, -7.856984441350959969 ) ) ;
#4816=ORIENTED_EDGE ( 'NONE', *, *, #427, .F. ) ;
#4823=ORIENTED_EDGE ( 'NONE', *, *, #9444, .F. ) ;
#4832=DIRECTION ( 'NONE',  ( 0.000000000000000000, 0.000000000000000000, 1.000000000000000000 ) ) ;
#4835=CARTESIAN_POINT ( 'NONE',  ( 8.373678438139048552, 0.000000000000000000, 1.459968977288628178 ) ) ;
#4836=ORIENTED_EDGE ( 'NONE', *, *, #9198, .F. ) ;
#4839=DIRECTION ( 'NONE',  ( 0.000000000000000000, 1.000000000000000000, -0.000000000000000000 ) ) ;
#4851=CIRCLE ( 'NONE', #6608, 8.499999999999996447 ) ;
#4861=CARTESIAN_POINT ( 'NONE',  ( 7.248474140376191421, 0.000000000000000000, 4.439552076088042476 ) ) ;
#4870=EDGE_CURVE ( 'NONE', #8226, #1004, #10368, .T. ) ;
#4878=CARTESIAN_POINT ( 'NONE',  ( 0.000000000000000000, 9.000000000000000000, 0.000000000000000000 ) ) ;
#4887=EDGE_LOOP ( 'NONE', ( #6159, #11460, #10997, #2414 ) ) ;
#4893=CARTESIAN_POINT ( 'NONE',  ( 7.248474140376192310, 9.000000000000000000, 4.439552076088041588 ) ) ;
#4897=CARTESIAN_POINT ( 'NONE',  ( -6.558450276537426404, 9.000000000000000000, -1.596630818375423866 ) ) ;
#4900=VECTOR ( 'NONE', #3721, 1000.000000000000000 ) ;
#4903=ORIENTED_EDGE ( 'NONE', *, *, #613, .F. ) ;
#4909=ORIENTED_EDGE ( 'NONE', *, *, #7920, .F. ) ;
#4916=CARTESIAN_POINT ( 'NONE',  ( -4.679611352264966051, 0.000000000000000000, -6.417326716594978997 ) ) ;
#4918=ADVANCED_FACE ( 'NONE', ( #1706 ), #663, .T. ) ;
#4919=CARTESIAN_POINT ( 'NONE',  ( -4.190859029938718727, -1.694065894508600678E-18, -6.054087828318142073 ) ) ;
#4928=ORIENTED_EDGE ( 'NONE', *, *, #11148, .F. ) ;
#4935=APPLICATION_CONTEXT ( 'automotive_design' ) ;
#4944=ORIENTED_EDGE ( 'NONE', *, *, #2697, .F. ) ;
#4946=ORIENTED_EDGE ( 'NONE', *, *, #7922, .T. ) ;
#4948=VERTEX_POINT ( 'NONE', #4370 ) ;
#4956=CARTESIAN_POINT ( 'NONE',  ( 0.000000000000000000, 9.000000000000000000, 0.000000000000000000 ) ) ;
#4957=CARTESIAN_POINT ( 'NONE',  ( 2.458659560121116527, 9.000000000000000000, -8.136645080586040635 ) ) ;
#4964=VECTOR ( 'NONE', #6460, 1000.000000000000000 ) ;
#4972=DIRECTION ( 'NONE',  ( -0.000000000000000000, -1.000000000000000000, -0.000000000000000000 ) ) ;
#4974=ORIENTED_EDGE ( 'NONE', *, *, #8509, .F. ) ;
#4980=CARTESIAN_POINT ( 'NONE',  ( -3.835481108877868195, 1.734723475976807094E-15, 5.554420281491219136 ) ) ;
#4985=FACE_OUTER_BOUND ( 'NONE', #4124, .T. ) ;
#4995=ORIENTED_EDGE ( 'NONE', *, *, #7755, .F. ) ;
#4998=EDGE_CURVE ( 'NONE', #12645, #9873, #3322, .T. ) ;
#5013=CARTESIAN_POINT ( 'NONE',  ( -2.481593227817850966, 0.000000000000000000, -8.129679886173169834 ) ) ;
#5038=ORIENTED_EDGE ( 'NONE', *, *, #7769, .F. ) ;
#5052=ORIENTED_EDGE ( 'NONE', *, *, #4467, .F. ) ;
#5067=DIRECTION ( 'NONE',  ( 0.000000000000000000, 1.000000000000000000, -0.000000000000000000 ) ) ;
#5080=EDGE_CURVE ( 'NONE', #1998, #2013, #3075, .T. ) ;
#5088=AXIS2_PLACEMENT_3D ( 'NONE', #6776, #5532, #11951 ) ;
#5094=ORIENTED_EDGE ( 'NONE', *, *, #6118, .F. ) ;
#5097=LINE ( 'NONE', #6070, #10070 ) ;
#5099=CARTESIAN_POINT ( 'NONE',  ( 0.000000000000000000, 9.000000000000000000, 0.000000000000000000 ) ) ;
#5104=CLOSED_SHELL ( 'NONE', ( #6346, #4729, #7772, #7160, #3135, #12424, #8929, #8413, #640, #5430, #8925, #7004, #1328, #10623, #7115, #5346, #10816, #10300, #5184, #10309, #4918, #2971, #1685, #5899, #10703, #6771, #9806, #4054, #8806, #6866, #7593, #3989, #3299, #2854, #3529, #191, #12368, #8709, #5860, #11629, #2451, #2115, #2718, #10301, #7955, #4225, #1216, #3536, #4315, #8125, #8577, #4643, #4006, #9240, #369, #9532, #7870, #11032, #4551, #4151, #4639 ) ) ;
#5107=ORIENTED_EDGE ( 'NONE', *, *, #8448, .F. ) ;
#5122=CARTESIAN_POINT ( 'NONE',  ( -8.100301009650792139, 9.000000000000000000, -2.575873357339267589 ) ) ;
#5123=ORIENTED_EDGE ( 'NONE', *, *, #10875, .F. ) ;
#5124=CARTESIAN_POINT ( 'NONE',  ( -8.369528376005813897, 9.000000000000000000, 1.483574994138650460 ) ) ;
#5128=CIRCLE ( 'NONE', #11284, 6.749999999999999112 ) ;
#5137=VECTOR ( 'NONE', #8908, 1000.000000000000000 ) ;
#5146=EDGE_CURVE ( 'NONE', #1296, #9824, #440, .T. ) ;
#5147=CARTESIAN_POINT ( 'NONE',  ( 6.749972395921142621, 0.000000000000000000, -0.01930425607464712062 ) ) ;
#5150=AXIS2_PLACEMENT_3D ( 'NONE', #12288, #2830, #6972 ) ;
#5152=CARTESIAN_POINT ( 'NONE',  ( 6.553553527263006551, 9.000000000000000000, 1.616612558808879774 ) ) ;
#5157=LINE ( 'NONE', #7425, #2437 ) ;
#5160=VECTOR ( 'NONE', #11493, 1000.000000000000000 ) ;
#5162=CARTESIAN_POINT ( 'NONE',  ( 5.051606143860418285, 0.000000000000000000, 4.477027514692275112 ) ) ;
#5174=CARTESIAN_POINT ( 'NONE',  ( -6.934601996837493232, 0.000000000000000000, 3.871968458191308748 ) ) ;
#5176=CARTESIAN_POINT ( 'NONE',  ( -3.533475733155563070, 9.000000000000000000, 7.730753471893976325 ) ) ;
#5184=ADVANCED_FACE ( 'NONE', ( #1548 ), #5739, .T. ) ;
#5185=ORIENTED_EDGE ( 'NONE', *, *, #6318, .F. ) ;
#5186=EDGE_CURVE ( 'NONE', #9762, #3498, #2829, .T. ) ;
#5190=CARTESIAN_POINT ( 'NONE',  ( -0.8973464813148227526, 9.000000000000000000, -7.308217849399443189 ) ) ;
#5193=CARTESIAN_POINT ( 'NONE',  ( 2.623034112301249721, 0.000000000000000000, -7.496701717520498853 ) ) ;
#5204=ORIENTED_EDGE ( 'NONE', *, *, #7702, .T. ) ;
#5212=ORIENTED_EDGE ( 'NONE', *, *, #7755, .T. ) ;
#5229=CARTESIAN_POINT ( 'NONE',  ( 4.355042381134426321, 9.000000000000000000, 7.299562031966228659 ) ) ;
#5233=DIRECTION ( 'NONE',  ( 0.000000000000000000, 0.000000000000000000, 1.000000000000000000 ) ) ;
#5237=CARTESIAN_POINT ( 'NONE',  ( 0.8653219153705552502, 9.000000000000000000, -7.312626806738413698 ) ) ;
#5239=VERTEX_POINT ( 'NONE', #8146 ) ;
#5243=VERTEX_POINT ( 'NONE', #8087 ) ;
#5244=B_SPLINE_CURVE_WITH_KNOTS ( 'NONE', 3,
 ( #1243, #3432, #6476, #11847 ),
 .UNSPECIFIED., .F., .F.,
 ( 4, 4 ),
 ( 0.000000000000000000, 0.8724294488011775650 ),
 .UNSPECIFIED. ) ;
#5253=CARTESIAN_POINT ( 'NONE',  ( -5.976238463952679325, 9.000000000000000000, -3.138004751744733589 ) ) ;
#5257=DIRECTION ( 'NONE',  ( 0.000000000000000000, 1.000000000000000000, -0.000000000000000000 ) ) ;
#5262=DIRECTION ( 'NONE',  ( 0.000000000000000000, 0.000000000000000000, 1.000000000000000000 ) ) ;
#5267=DIRECTION ( 'NONE',  ( -0.000000000000000000, -1.000000000000000000, -0.000000000000000000 ) ) ;
#5271=ORIENTED_EDGE ( 'NONE', *, *, #490, .F. ) ;
#5274=B_SPLINE_CURVE_WITH_KNOTS ( 'NONE', 3,
 ( #12973, #5804, #5601, #10006 ),
 .UNSPECIFIED., .F., .F.,
 ( 4, 4 ),
 ( 0.000000000000000000, 0.8724294488011774540 ),
 .UNSPECIFIED. ) ;
#5289=ORIENTED_EDGE ( 'NONE', *, *, #8235, .F. ) ;
#5312=EDGE_CURVE ( 'NONE', #7170, #2755, #7281, .T. ) ;
#5320=DIRECTION ( 'NONE',  ( 0.000000000000000000, 0.000000000000000000, 1.000000000000000000 ) ) ;
#5325=ORIENTED_EDGE ( 'NONE', *, *, #4748, .F. ) ;
#5332=CARTESIAN_POINT ( 'NONE',  ( -5.065227977808753224, 9.000000000000000000, -4.461610195077944319 ) ) ;
#5334=B_SPLINE_CURVE_WITH_KNOTS ( 'NONE', 3,
 ( #11181, #13046, #1544, #8081 ),
 .UNSPECIFIED., .F., .F.,
 ( 4, 4 ),
 ( 0.000000000000000000, 0.8724294488011774540 ),
 .UNSPECIFIED. ) ;
#5341=AXIS2_PLACEMENT_3D ( 'NONE', #6156, #5257, #2925 ) ;
#5342=VERTEX_POINT ( 'NONE', #13536 ) ;
#5346=ADVANCED_FACE ( 'NONE', ( #3364 ), #3443, .T. ) ;
#5347=ORIENTED_EDGE ( 'NONE', *, *, #11545, .T. ) ;
#5358=AXIS2_PLACEMENT_3D ( 'NONE', #12945, #1172, #1301 ) ;
#5370=CARTESIAN_POINT ( 'NONE',  ( -8.100301009650799244, 9.000000000000000000, -2.575873357339268033 ) ) ;
#5375=LINE ( 'NONE', #6611, #9954 ) ;
#5390=CARTESIAN_POINT ( 'NONE',  ( -5.975392301194330180, 9.000000000000000000, -6.045220165289885372 ) ) ;
#5395=CARTESIAN_POINT ( 'NONE',  ( 3.555260608155774271, 9.000000000000000000, 7.720759160088842776 ) ) ;
#5399=ORIENTED_EDGE ( 'NONE', *, *, #11804, .T. ) ;
#5402=CARTESIAN_POINT ( 'NONE',  ( -6.749999880766614169, 9.000000000000000000, -0.001268720102703522860 ) ) ;
#5408=ORIENTED_EDGE ( 'NONE', *, *, #6581, .T. ) ;
#5430=ADVANCED_FACE ( 'NONE', ( #13117 ), #6412, .T. ) ;
#5439=ORIENTED_EDGE ( 'NONE', *, *, #535, .F. ) ;
#5442=DIRECTION ( 'NONE',  ( 0.000000000000000000, 0.000000000000000000, -1.000000000000000000 ) ) ;
#5456=ORIENTED_EDGE ( 'NONE', *, *, #11051, .F. ) ;
#5457=EDGE_LOOP ( 'NONE', ( #13400, #11668, #7878, #3658 ) ) ;
#5466=CARTESIAN_POINT ( 'NONE',  ( 0.9098489087730803337, 0.000000000000000000, 7.307220250892556557 ) ) ;
#5468=EDGE_LOOP ( 'NONE', ( #10276, #3039, #8065, #4243 ) ) ;
#5469=CARTESIAN_POINT ( 'NONE',  ( 4.201465772524378472, 0.000000000000000000, 6.047394330962382547 ) ) ;
#5478=LINE ( 'NONE', #5623, #13215 ) ;
#5497=CARTESIAN_POINT ( 'NONE',  ( -7.155006492985575228, 9.000000000000000000, -1.740452503570284915 ) ) ;
#5498=DIRECTION ( 'NONE',  ( 0.000000000000000000, 1.000000000000000000, -0.000000000000000000 ) ) ;
#5501=DIRECTION ( 'NONE',  ( -0.000000000000000000, -1.000000000000000000, -0.000000000000000000 ) ) ;
#5509=EDGE_LOOP ( 'NONE', ( #729, #4903, #13508, #6129 ) ) ;
#5512=SHAPE_REPRESENTATION_RELATIONSHIP ( 'NONE' , 'NONE' ,  #8376, #10000 ) ;
#5516=DIRECTION ( 'NONE',  ( 0.000000000000000000, 0.000000000000000000, -1.000000000000000000 ) ) ;
#5519=ORIENTED_EDGE ( 'NONE', *, *, #2119, .T. ) ;
#5522=AXIS2_PLACEMENT_3D ( 'NONE', #13259, #13051, #10015 ) ;
#5526=ORIENTED_EDGE ( 'NONE', *, *, #2184, .F. ) ;
#5527=CARTESIAN_POINT ( 'NONE',  ( 8.373678438139048552, 9.000000000000000000, 1.459968977288628844 ) ) ;
#5532=DIRECTION ( 'NONE',  ( 0.000000000000000000, 1.000000000000000000, -0.000000000000000000 ) ) ;
#5560=ORIENTED_EDGE ( 'NONE', *, *, #2619, .F. ) ;
#5564=LINE ( 'NONE', #4538, #13190 ) ;
#5565=CARTESIAN_POINT ( 'NONE',  ( 6.736042615721505200, 9.000000000000000000, 5.184180733653466433 ) ) ;
#5575=DIRECTION ( 'NONE',  ( -0.000000000000000000, -1.000000000000000000, -0.000000000000000000 ) ) ;
#5593=CARTESIAN_POINT ( 'NONE',  ( -4.334442004268530546, 9.000000000000000000, 7.311813216407585081 ) ) ;
#5601=CARTESIAN_POINT ( 'NONE',  ( 6.951477219042924816, 9.000000000000000000, 3.842108769784387423 ) ) ;
#5606=CARTESIAN_POINT ( 'NONE',  ( 6.749972395921142621, 0.000000000000000000, -0.01930425607464666612 ) ) ;
#5609=CARTESIAN_POINT ( 'NONE',  ( 6.553553527263006551, 1.734723475976807094E-15, 1.616612558808879774 ) ) ;
#5611=DIRECTION ( 'NONE',  ( 0.000000000000000000, 1.000000000000000000, -0.000000000000000000 ) ) ;
#5612=VERTEX_POINT ( 'NONE', #2023 ) ;
#5615=VERTEX_POINT ( 'NONE', #11255 ) ;
#5623=CARTESIAN_POINT ( 'NONE',  ( 5.280889752749253319, 9.000000000000000000, -6.660495733750448011 ) ) ;
#5633=EDGE_CURVE ( 'NONE', #8226, #5615, #10225, .T. ) ;
#5634=CYLINDRICAL_SURFACE ( 'NONE', #10328, 6.750000000000000888 ) ;
#5653=CARTESIAN_POINT ( 'NONE',  ( 0.9098489087730803337, 0.000000000000000000, 7.307220250892556557 ) ) ;
#5670=CARTESIAN_POINT ( 'NONE',  ( -7.751044794789887504, 0.000000000000000000, 1.733822342365972879 ) ) ;
#5673=CARTESIAN_POINT ( 'NONE',  ( 0.7868956173019259204, 0.000000000000000000, 7.903520140620750034 ) ) ;
#5677=EDGE_CURVE ( 'NONE', #2261, #3196, #6441, .T. ) ;
#5683=CARTESIAN_POINT ( 'NONE',  ( 4.164551629694410728, 0.000000000000000000, -6.072874324029720050 ) ) ;
#5690=ORIENTED_EDGE ( 'NONE', *, *, #2196, .F. ) ;
#5694=VERTEX_POINT ( 'NONE', #2604 ) ;
#5707=EDGE_LOOP ( 'NONE', ( #12309, #7371, #4777, #9492 ) ) ;
#5712=DIRECTION ( 'NONE',  ( 1.000000000000000000, 0.000000000000000000, 0.000000000000000000 ) ) ;
#5727=VECTOR ( 'NONE', #7685, 1000.000000000000000 ) ;
#5739=CYLINDRICAL_SURFACE ( 'NONE', #915, 8.500000000000000000 ) ;
#5740=DIRECTION ( 'NONE',  ( -0.000000000000000000, -1.000000000000000000, -0.000000000000000000 ) ) ;
#5751=FACE_OUTER_BOUND ( 'NONE', #9189, .T. ) ;
#5754=CARTESIAN_POINT ( 'NONE',  ( 6.951477219042924816, 0.000000000000000000, 3.842108769784387423 ) ) ;
#5759=CARTESIAN_POINT ( 'NONE',  ( 0.000000000000000000, 9.000000000000000000, 0.000000000000000000 ) ) ;
#5762=ORIENTED_EDGE ( 'NONE', *, *, #7710, .F. ) ;
#5771=B_SPLINE_SURFACE_WITH_KNOTS ( 'NONE', 3, 1, ( 
 ( #6125, #10188 ),
 ( #9289, #9217 ),
 ( #13567, #8256 ),
 ( #766, #5162 ) ),
 .UNSPECIFIED., .F., .F., .F.,
 ( 4, 4 ),
 ( 2, 2 ),
 ( 0.1276832474596250877, 1.000000000000000000 ),
 ( 0.000000000000000000, 1.000000000000000000 ),
 .UNSPECIFIED. ) ;
#5772=CARTESIAN_POINT ( 'NONE',  ( 0.000000000000000000, 9.000000000000000000, 0.000000000000000000 ) ) ;
#5776=FACE_OUTER_BOUND ( 'NONE', #398, .T. ) ;
#5786=CARTESIAN_POINT ( 'NONE',  ( 1.127406311874972422, 9.000000000000000000, -7.862174656777307646 ) ) ;
#5791=FACE_OUTER_BOUND ( 'NONE', #8139, .T. ) ;
#5793=EDGE_CURVE ( 'NONE', #75, #6767, #1337, .T. ) ;
#5798=CARTESIAN_POINT ( 'NONE',  ( -0.4399887592034530392, 9.000000000000000000, 8.488604708182295511 ) ) ;
#5802=CIRCLE ( 'NONE', #7352, 6.750000000000001776 ) ;
#5804=CARTESIAN_POINT ( 'NONE',  ( 6.530577460941774603, 9.000000000000000000, 3.402183248810843885 ) ) ;
#5819=CARTESIAN_POINT ( 'NONE',  ( 5.967832595844252630, 9.000000000000000000, -3.153961652902406154 ) ) ;
#5822=ORIENTED_EDGE ( 'NONE', *, *, #5080, .F. ) ;
#5823=MECHANICAL_DESIGN_GEOMETRIC_PRESENTATION_REPRESENTATION('',(#11764),#11108);
#5826=CARTESIAN_POINT ( 'NONE',  ( -3.533475733155563070, 0.000000000000000000, 7.730753471893976325 ) ) ;
#5829=CARTESIAN_POINT ( 'NONE',  ( 0.000000000000000000, 9.000000000000000000, 0.000000000000000000 ) ) ;
#5831=MECHANICAL_DESIGN_GEOMETRIC_PRESENTATION_REPRESENTATION('',(#11998),#7598);
#5839=VERTEX_POINT ( 'NONE', #3908 ) ;
#5847=CARTESIAN_POINT ( 'NONE',  ( -6.721397655168936502, 0.000000000000000000, 5.203154193476255074 ) ) ;
#5848=CARTESIAN_POINT ( 'NONE',  ( 5.985774866078160450, 9.000000000000000000, 3.119775513178307147 ) ) ;
#5854=DIRECTION ( 'NONE',  ( -0.000000000000000000, -1.000000000000000000, -0.000000000000000000 ) ) ;
#5858=EDGE_LOOP ( 'NONE', ( #7010, #5038, #7099, #8586 ) ) ;
#5860=ADVANCED_FACE ( 'NONE', ( #4750 ), #11152, .T. ) ;
#5866=CARTESIAN_POINT ( 'NONE',  ( 5.051606143860416509, 9.000000000000000000, 4.477027514692274224 ) ) ;
#5874=CARTESIAN_POINT ( 'NONE',  ( 7.758214145541979967, -1.694065894508600678E-18, 1.700281702449083054 ) ) ;
#5876=B_SPLINE_SURFACE_WITH_KNOTS ( 'NONE', 3, 1, ( 
 ( #3978, #8178 ),
 ( #7898, #10106 ),
 ( #12121, #2671 ),
 ( #1657, #5847 ) ),
 .UNSPECIFIED., .F., .F., .F.,
 ( 4, 4 ),
 ( 2, 2 ),
 ( 0.000000000000000000, 0.8724294488011775650 ),
 ( 0.000000000000000000, 1.000000000000000000 ),
 .UNSPECIFIED. ) ;
#5890=VERTEX_POINT ( 'NONE', #3696 ) ;
#5896=DIRECTION ( 'NONE',  ( 0.000000000000000000, 1.000000000000000000, -0.000000000000000000 ) ) ;
#5897=CYLINDRICAL_SURFACE ( 'NONE', #11077, 8.499999999999996447 ) ;
#5899=ADVANCED_FACE ( 'NONE', ( #9211 ), #5876, .T. ) ;
#5904=ORIENTED_EDGE ( 'NONE', *, *, #2322, .T. ) ;
#5909=DIRECTION ( 'NONE',  ( 0.000000000000000000, 1.000000000000000000, -0.000000000000000000 ) ) ;
#5914=ORIENTED_EDGE ( 'NONE', *, *, #1276, .T. ) ;
#5918=VERTEX_POINT ( 'NONE', #10465 ) ;
#5922=EDGE_CURVE ( 'NONE', #10329, #11033, #12780, .T. ) ;
#5925=B_SPLINE_CURVE_WITH_KNOTS ( 'NONE', 3,
 ( #10245, #9056, #7006, #743 ),
 .UNSPECIFIED., .F., .F.,
 ( 4, 4 ),
 ( 0.000000000000000000, 0.8724294488011762327 ),
 .UNSPECIFIED. ) ;
#5928=CARTESIAN_POINT ( 'NONE',  ( 0.4639228963249704130, 9.000000000000000000, 8.487330295579726069 ) ) ;
#5938=LINE ( 'NONE', #3800, #12817 ) ;
#5939=EDGE_LOOP ( 'NONE', ( #1438, #5123, #8023, #6357 ) ) ;
#5945=DIRECTION ( 'NONE',  ( 0.000000000000000000, 1.000000000000000000, -0.000000000000000000 ) ) ;
#5947=CARTESIAN_POINT ( 'NONE',  ( 0.7868956173019259204, 9.000000000000000000, 7.903520140620750034 ) ) ;
#5957=ORIENTED_EDGE ( 'NONE', *, *, #2184, .T. ) ;
#5960=AXIS2_PLACEMENT_3D ( 'NONE', #3080, #1155, #9285 ) ;
#5965=EDGE_CURVE ( 'NONE', #9600, #10417, #5157, .T. ) ;
#5990=ORIENTED_EDGE ( 'NONE', *, *, #9541, .T. ) ;
#5994=ORIENTED_EDGE ( 'NONE', *, *, #44, .F. ) ;
#6013=DIRECTION ( 'NONE',  ( 0.000000000000000000, 0.000000000000000000, -1.000000000000000000 ) ) ;
#6019=( NAMED_UNIT ( * ) PLANE_ANGLE_UNIT ( ) SI_UNIT ( $, .RADIAN. ) );
#6024=CARTESIAN_POINT ( 'NONE',  ( -0.4399887592034530392, 9.000000000000000000, 8.488604708182295511 ) ) ;
#6032=ORIENTED_EDGE ( 'NONE', *, *, #8274, .T. ) ;
#6039=VECTOR ( 'NONE', #9563, 1000.000000000000000 ) ;
#6043=AXIS2_PLACEMENT_3D ( 'NONE', #1818, #9241, #1953 ) ;
#6046=CARTESIAN_POINT ( 'NONE',  ( 0.000000000000000000, 0.000000000000000000, 0.000000000000000000 ) ) ;
#6056=B_SPLINE_CURVE_WITH_KNOTS ( 'NONE', 3,
 ( #13052, #5466, #5673, #248 ),
 .UNSPECIFIED., .F., .F.,
 ( 4, 4 ),
 ( 0.000000000000000000, 0.8724294488011784532 ),
 .UNSPECIFIED. ) ;
#6062=CARTESIAN_POINT ( 'NONE',  ( -5.976238463952679325, 0.000000000000000000, -3.138004751744733589 ) ) ;
#6064=FACE_OUTER_BOUND ( 'NONE', #771, .T. ) ;
#6070=CARTESIAN_POINT ( 'NONE',  ( -5.039625798601655937, 9.000000000000000000, 4.490509081392509927 ) ) ;
#6071=CARTESIAN_POINT ( 'NONE',  ( 0.000000000000000000, 9.000000000000000000, 0.000000000000000000 ) ) ;
#6072=DIRECTION ( 'NONE',  ( 0.000000000000000000, 0.000000000000000000, -1.000000000000000000 ) ) ;
#6082=EDGE_CURVE ( 'NONE', #1535, #6548, #456, .T. ) ;
#6088=EDGE_CURVE ( 'NONE', #12927, #9922, #5478, .T. ) ;
#6094=CARTESIAN_POINT ( 'NONE',  ( 5.280889752749253319, 0.000000000000000000, -6.660495733750448899 ) ) ;
#6108=FACE_OUTER_BOUND ( 'NONE', #5468, .T. ) ;
#6114=LINE ( 'NONE', #10313, #11040 ) ;
#6118=EDGE_CURVE ( 'NONE', #7648, #6374, #12574, .T. ) ;
#6125=CARTESIAN_POINT ( 'NONE',  ( 6.736042615721505200, 9.000000000000000000, 5.184180733653466433 ) ) ;
#6126=ORIENTED_EDGE ( 'NONE', *, *, #2285, .F. ) ;
#6129=ORIENTED_EDGE ( 'NONE', *, *, #9444, .T. ) ;
#6141=CARTESIAN_POINT ( 'NONE',  ( 2.458659560121116527, 9.000000000000000000, -8.136645080586040635 ) ) ;
#6152=CARTESIAN_POINT ( 'NONE',  ( -3.835481108877868195, 9.000000000000000000, 5.554420281491219136 ) ) ;
#6156=CARTESIAN_POINT ( 'NONE',  ( 0.000000000000000000, 9.000000000000000000, 0.000000000000000000 ) ) ;
#6157=ORIENTED_EDGE ( 'NONE', *, *, #4327, .F. ) ;
#6159=ORIENTED_EDGE ( 'NONE', *, *, #6118, .T. ) ;
#6161=AXIS2_PLACEMENT_3D ( 'NONE', #10725, #5945, #4710 ) ;
#6162=ORIENTED_EDGE ( 'NONE', *, *, #2207, .F. ) ;
#6163=ORIENTED_EDGE ( 'NONE', *, *, #12652, .F. ) ;
#6172=DIRECTION ( 'NONE',  ( 0.000000000000000000, 0.000000000000000000, 1.000000000000000000 ) ) ;
#6178=AXIS2_PLACEMENT_3D ( 'NONE', #5772, #10803, #13084 ) ;
#6196=CARTESIAN_POINT ( 'NONE',  ( 2.392396671352951198, 0.000000000000000000, 6.311809420990095454 ) ) ;
#6204=ORIENTED_EDGE ( 'NONE', *, *, #3752, .T. ) ;
#6217=VECTOR ( 'NONE', #12145, 1000.000000000000000 ) ;
#6221=CARTESIAN_POINT ( 'NONE',  ( 4.652003457867571967, 0.000000000000000000, -6.437678087145717321 ) ) ;
#6231=ORIENTED_EDGE ( 'NONE', *, *, #321, .T. ) ;
#6250=EDGE_CURVE ( 'NONE', #5694, #11681, #5925, .T. ) ;
#6267=CARTESIAN_POINT ( 'NONE',  ( 6.553553527263006551, 9.000000000000000000, 1.616612558808879774 ) ) ;
#6268=CARTESIAN_POINT ( 'NONE',  ( 0.000000000000000000, 9.000000000000000000, 0.000000000000000000 ) ) ;
#6270=FACE_OUTER_BOUND ( 'NONE', #4432, .T. ) ;
#6275=ORIENTED_EDGE ( 'NONE', *, *, #8265, .F. ) ;
#6279=EDGE_CURVE ( 'NONE', #5890, #5239, #12675, .T. ) ;
#6280=ORIENTED_EDGE ( 'NONE', *, *, #6088, .T. ) ;
#6303=B_SPLINE_CURVE_WITH_KNOTS ( 'NONE', 3,
 ( #9933, #11186, #5947, #1691 ),
 .UNSPECIFIED., .F., .F.,
 ( 4, 4 ),
 ( 0.000000000000000000, 0.8724294488011784532 ),
 .UNSPECIFIED. ) ;
#6318=EDGE_CURVE ( 'NONE', #10298, #7353, #6410, .T. ) ;
#6320=EDGE_CURVE ( 'NONE', #11737, #3918, #1344, .T. ) ;
#6325=ORIENTED_EDGE ( 'NONE', *, *, #10350, .T. ) ;
#6334=B_SPLINE_CURVE_WITH_KNOTS ( 'NONE', 3,
 ( #3237, #7511, #2348, #7709 ),
 .UNSPECIFIED., .F., .F.,
 ( 4, 4 ),
 ( 0.000000000000000000, 0.8724294488011776760 ),
 .UNSPECIFIED. ) ;
#6336=PRODUCT_DEFINITION_SHAPE ( 'NONE', 'NONE',  #10940 ) ;
#6346=ADVANCED_FACE ( 'NONE', ( #6108 ), #7151, .T. ) ;
#6352=CARTESIAN_POINT ( 'NONE',  ( -7.125870497355421662, 9.000000000000000000, -3.507536778237742237 ) ) ;
#6354=CARTESIAN_POINT ( 'NONE',  ( -0.4399887592034473771, 0.000000000000000000, 8.488604708182295511 ) ) ;
#6356=CARTESIAN_POINT ( 'NONE',  ( 6.736042615721505200, 0.000000000000000000, 5.184180733653466433 ) ) ;
#6357=ORIENTED_EDGE ( 'NONE', *, *, #4597, .T. ) ;
#6364=CARTESIAN_POINT ( 'NONE',  ( 3.850308450823737516, 0.000000000000000000, 5.544152309732777617 ) ) ;
#6374=VERTEX_POINT ( 'NONE', #11349 ) ;
#6379=FACE_OUTER_BOUND ( 'NONE', #3420, .T. ) ;
#6385=EDGE_LOOP ( 'NONE', ( #13374, #7635, #1711, #2178 ) ) ;
#6395=CIRCLE ( 'NONE', #5522, 6.750000000000000888 ) ;
#6396=DIRECTION ( 'NONE',  ( 0.000000000000000000, 0.000000000000000000, -1.000000000000000000 ) ) ;
#6409=AXIS2_PLACEMENT_3D ( 'NONE', #1304, #5498, #9703 ) ;
#6410=B_SPLINE_CURVE_WITH_KNOTS ( 'NONE', 3,
 ( #4733, #8920, #7883, #12105 ),
 .UNSPECIFIED., .F., .F.,
 ( 4, 4 ),
 ( 0.1276832474596270861, 1.000000000000000000 ),
 .UNSPECIFIED. ) ;
#6412=B_SPLINE_SURFACE_WITH_KNOTS ( 'NONE', 3, 1, ( 
 ( #13255, #12089 ),
 ( #3667, #4916 ),
 ( #11121, #6773 ),
 ( #13334, #1689 ) ),
 .UNSPECIFIED., .F., .F., .F.,
 ( 4, 4 ),
 ( 2, 2 ),
 ( 0.1276832474596281686, 1.000000000000000000 ),
 ( 0.000000000000000000, 1.000000000000000000 ),
 .UNSPECIFIED. ) ;
#6417=LINE ( 'NONE', #4419, #9230 ) ;
#6419=AXIS2_PLACEMENT_3D ( 'NONE', #9273, #3967, #1981 ) ;
#6425=CARTESIAN_POINT ( 'NONE',  ( 8.373678438139048552, 0.000000000000000000, 1.459968977288628178 ) ) ;
#6427=CARTESIAN_POINT ( 'NONE',  ( 5.053288777954491273, 9.000000000000000000, -4.475128213425755952 ) ) ;
#6432=AXIS2_PLACEMENT_3D ( 'NONE', #10136, #12149, #6013 ) ;
#6433=CIRCLE ( 'NONE', #8833, 8.499999999999998224 ) ;
#6436=CARTESIAN_POINT ( 'NONE',  ( -6.515098946627274401, 9.000000000000000000, 3.430563300314522390 ) ) ;
#6441=B_SPLINE_CURVE_WITH_KNOTS ( 'NONE', 3,
 ( #4211, #6739, #3187, #6492 ),
 .UNSPECIFIED., .F., .F.,
 ( 4, 4 ),
 ( 0.000000000000000000, 0.8724294488011762327 ),
 .UNSPECIFIED. ) ;
#6442=CIRCLE ( 'NONE', #7332, 8.500000000000000000 ) ;
#6444=AXIS2_PLACEMENT_3D ( 'NONE', #6071, #11892, #454 ) ;
#6446=EDGE_LOOP ( 'NONE', ( #9569, #8187, #10621, #542 ) ) ;
#6452=DIRECTION ( 'NONE',  ( 0.000000000000000000, 0.000000000000000000, -1.000000000000000000 ) ) ;
#6458=DIRECTION ( 'NONE',  ( 0.000000000000000000, 1.000000000000000000, -0.000000000000000000 ) ) ;
#6460=DIRECTION ( 'NONE',  ( -0.000000000000000000, -1.000000000000000000, -0.000000000000000000 ) ) ;
#6466=ORIENTED_EDGE ( 'NONE', *, *, #2619, .T. ) ;
#6469=DIRECTION ( 'NONE',  ( 0.000000000000000000, 1.000000000000000000, -0.000000000000000000 ) ) ;
#6476=CARTESIAN_POINT ( 'NONE',  ( -6.057461899949976747, 9.000000000000000000, 5.137313564148215939 ) ) ;
#6485=VECTOR ( 'NONE', #3052, 1000.000000000000000 ) ;
#6492=CARTESIAN_POINT ( 'NONE',  ( -2.481593227817850966, 0.000000000000000000, -8.129679886173169834 ) ) ;
#6493=( GEOMETRIC_REPRESENTATION_CONTEXT ( 3 ) GLOBAL_UNCERTAINTY_ASSIGNED_CONTEXT ( ( #896 ) ) GLOBAL_UNIT_ASSIGNED_CONTEXT ( ( #12069, #13102, #2561 ) ) REPRESENTATION_CONTEXT ( 'NONE', 'WORKASPACE' ) );
#6501=EDGE_LOOP ( 'NONE', ( #4239, #9424, #7478, #3519 ) ) ;
#6508=CARTESIAN_POINT ( 'NONE',  ( 2.394769219159762930, 1.734723475976807094E-15, -6.310909632292713844 ) ) ;
#6516=ORIENTED_EDGE ( 'NONE', *, *, #12652, .T. ) ;
#6520=CARTESIAN_POINT ( 'NONE',  ( 0.000000000000000000, 0.000000000000000000, 0.000000000000000000 ) ) ;
#6525=DIRECTION ( 'NONE',  ( -0.000000000000000000, -1.000000000000000000, -0.000000000000000000 ) ) ;
#6526=EDGE_CURVE ( 'NONE', #11178, #2755, #3404, .T. ) ;
#6544=DIRECTION ( 'NONE',  ( 0.000000000000000000, 1.000000000000000000, -0.000000000000000000 ) ) ;
#6548=VERTEX_POINT ( 'NONE', #5609 ) ;
#6549=ORIENTED_EDGE ( 'NONE', *, *, #6526, .T. ) ;
#6560=LINE ( 'NONE', #5390, #924 ) ;
#6567=CARTESIAN_POINT ( 'NONE',  ( 7.758214145541979967, 0.000000000000000000, 1.700281702449083054 ) ) ;
#6571=CARTESIAN_POINT ( 'NONE',  ( -7.751044794789887504, 9.000000000000000000, 1.733822342365972879 ) ) ;
#6576=ORIENTED_EDGE ( 'NONE', *, *, #12994, .F. ) ;
#6581=EDGE_CURVE ( 'NONE', #12363, #7170, #3881, .T. ) ;
#6584=DIRECTION ( 'NONE',  ( 0.000000000000000000, -0.000000000000000000, -1.000000000000000000 ) ) ;
#6608=AXIS2_PLACEMENT_3D ( 'NONE', #6268, #2263, #5233 ) ;
#6611=CARTESIAN_POINT ( 'NONE',  ( 8.481367827640703183, 9.000000000000000000, 0.5624942419805127880 ) ) ;
#6614=ORIENTED_EDGE ( 'NONE', *, *, #737, .T. ) ;
#6617=AXIS2_PLACEMENT_3D ( 'NONE', #200, #6458, #8775 ) ;
#6620=EDGE_CURVE ( 'NONE', #10761, #11792, #6395, .T. ) ;
#6622=SURFACE_STYLE_FILL_AREA ( #569 ) ;
#6627=CARTESIAN_POINT ( 'NONE',  ( -4.174571361198896824, 9.000000000000000000, 6.065330394303907191 ) ) ;
#6628=ORIENTED_EDGE ( 'NONE', *, *, #1343, .F. ) ;
#6634=CARTESIAN_POINT ( 'NONE',  ( -0.8776997859584816375, 9.000000000000000000, 7.310603390113379341 ) ) ;
#6636=CIRCLE ( 'NONE', #10157, 8.500000000000000000 ) ;
#6638=CARTESIAN_POINT ( 'NONE',  ( -8.479748006907129820, 9.000000000000000000, 0.5864074857593144507 ) ) ;
#6649=B_SPLINE_SURFACE_WITH_KNOTS ( 'NONE', 3, 1, ( 
 ( #7326, #4018 ),
 ( #6352, #11529 ),
 ( #2093, #1056 ),
 ( #5253, #3189 ) ),
 .UNSPECIFIED., .F., .F., .F.,
 ( 4, 4 ),
 ( 2, 2 ),
 ( 0.1276832474596248101, 1.000000000000000000 ),
 ( 0.000000000000000000, 1.000000000000000000 ),
 .UNSPECIFIED. ) ;
#6651=DIRECTION ( 'NONE',  ( 0.000000000000000000, 1.000000000000000000, -0.000000000000000000 ) ) ;
#6659=CARTESIAN_POINT ( 'NONE',  ( 6.530577460941774603, 0.000000000000000000, 3.402183248810843885 ) ) ;
#6661=DIRECTION ( 'NONE',  ( 0.000000000000000000, 0.000000000000000000, -1.000000000000000000 ) ) ;
#6674=EDGE_CURVE ( 'NONE', #7910, #3196, #12305, .T. ) ;
#6675=B_SPLINE_CURVE_WITH_KNOTS ( 'NONE', 3,
 ( #5147, #8167, #4043, #8107 ),
 .UNSPECIFIED., .F., .F.,
 ( 4, 4 ),
 ( 0.000000000000000000, 0.8724294488011776760 ),
 .UNSPECIFIED. ) ;
#6678=VECTOR ( 'NONE', #256, 1000.000000000000000 ) ;
#6679=CARTESIAN_POINT ( 'NONE',  ( -4.334442004268530546, 9.000000000000000000, 7.311813216407585081 ) ) ;
#6686=PRODUCT_DEFINITION_CONTEXT ( 'detailed design', #10569, 'design' ) ;
#6689=ORIENTED_EDGE ( 'NONE', *, *, #7250, .F. ) ;
#6691=AXIS2_PLACEMENT_3D ( 'NONE', #7657, #1321, #5516 ) ;
#6714=CARTESIAN_POINT ( 'NONE',  ( 0.8327827707325454742, 9.000000000000000000, 6.698430626405788679 ) ) ;
#6723=CARTESIAN_POINT ( 'NONE',  ( 0.000000000000000000, -3.000000000000000000, 0.000000000000000000 ) ) ;
#6734=ORIENTED_EDGE ( 'NONE', *, *, #1796, .T. ) ;
#6735=B_SPLINE_CURVE_WITH_KNOTS ( 'NONE', 3,
 ( #6364, #10572, #1135, #1540 ),
 .UNSPECIFIED., .F., .F.,
 ( 4, 4 ),
 ( 0.000000000000000000, 0.8724294488011777871 ),
 .UNSPECIFIED. ) ;
#6739=CARTESIAN_POINT ( 'NONE',  ( -2.632142621505047408, 0.000000000000000000, -6.877144614729746586 ) ) ;
#6754=CARTESIAN_POINT ( 'NONE',  ( 0.000000000000000000, 0.000000000000000000, 0.000000000000000000 ) ) ;
#6755=CARTESIAN_POINT ( 'NONE',  ( -7.235926821844430812, 0.000000000000000000, 4.459973433655439301 ) ) ;
#6765=ORIENTED_EDGE ( 'NONE', *, *, #8055, .T. ) ;
#6767=VERTEX_POINT ( 'NONE', #9327 ) ;
#6768=CARTESIAN_POINT ( 'NONE',  ( -7.939678587550617728, -1.694065894508600678E-18, 0.2057875656132798770 ) ) ;
#6771=ADVANCED_FACE ( 'NONE', ( #9248 ), #9095, .T. ) ;
#6773=CARTESIAN_POINT ( 'NONE',  ( -4.190859029938718727, 0.000000000000000000, -6.054087828318142073 ) ) ;
#6776=CARTESIAN_POINT ( 'NONE',  ( 0.000000000000000000, 0.000000000000000000, 0.000000000000000000 ) ) ;
#6777=CARTESIAN_POINT ( 'NONE',  ( -2.481593227817846525, 9.000000000000000000, -8.129679886173168057 ) ) ;
#6781=ORIENTED_EDGE ( 'NONE', *, *, #2285, .T. ) ;
#6811=CARTESIAN_POINT ( 'NONE',  ( -2.375523406013128724, 9.000000000000000000, 6.318179211409233886 ) ) ;
#6815=VERTEX_POINT ( 'NONE', #7203 ) ;
#6826=CARTESIAN_POINT ( 'NONE',  ( 6.079397157347990799, 9.000000000000000000, 5.110946565852551693 ) ) ;
#6836=EDGE_CURVE ( 'NONE', #3870, #10809, #6560, .T. ) ;
#6837=CARTESIAN_POINT ( 'NONE',  ( 0.000000000000000000, 9.000000000000000000, 0.000000000000000000 ) ) ;
#6850=ORIENTED_EDGE ( 'NONE', *, *, #3263, .F. ) ;
#6853=ORIENTED_EDGE ( 'NONE', *, *, #4470, .T. ) ;
#6862=FACE_OUTER_BOUND ( 'NONE', #2300, .T. ) ;
#6866=ADVANCED_FACE ( 'NONE', ( #1125 ), #3389, .T. ) ;
#6868=CARTESIAN_POINT ( 'NONE',  ( -1.604252589105048976, 9.000000000000000000, -8.347237484961699039 ) ) ;
#6870=AXIS2_PLACEMENT_3D ( 'NONE', #12629, #3302, #12698 ) ;
#6888=CARTESIAN_POINT ( 'NONE',  ( -8.100301009650799244, 0.000000000000000000, -2.575873357339268033 ) ) ;
#6894=CARTESIAN_POINT ( 'NONE',  ( -5.977417671213807182, 1.734723475976807094E-15, 3.135757960025121527 ) ) ;
#6901=CARTESIAN_POINT ( 'NONE',  ( 5.051606143860416509, 9.000000000000000000, 4.477027514692274224 ) ) ;
#6905=CARTESIAN_POINT ( 'NONE',  ( -4.334442004268530546, 0.000000000000000000, 7.311813216407585081 ) ) ;
#6947=B_SPLINE_CURVE_WITH_KNOTS ( 'NONE', 3,
 ( #407, #1658, #10047, #1580 ),
 .UNSPECIFIED., .F., .F.,
 ( 4, 4 ),
 ( 0.000000000000000000, 0.8724294488011758997 ),
 .UNSPECIFIED. ) ;
#6959=ORIENTED_EDGE ( 'NONE', *, *, #8463, .F. ) ;
#6962=UNCERTAINTY_MEASURE_WITH_UNIT (LENGTH_MEASURE( 1.000000000000000082E-05 ), #2357, 'distance_accuracy_value', 'NONE');
#6964=CARTESIAN_POINT ( 'NONE',  ( -2.590203375110137873, 9.000000000000000000, 6.893050072893555758 ) ) ;
#6970=CARTESIAN_POINT ( 'NONE',  ( 0.000000000000000000, 9.000000000000000000, 0.000000000000000000 ) ) ;
#6972=DIRECTION ( 'NONE',  ( 0.000000000000000000, 0.000000000000000000, -1.000000000000000000 ) ) ;
#6975=ORIENTED_EDGE ( 'NONE', *, *, #7064, .T. ) ;
#6977=ORIENTED_EDGE ( 'NONE', *, *, #3411, .T. ) ;
#6985=DIRECTION ( 'NONE',  ( 0.000000000000000000, 0.000000000000000000, 1.000000000000000000 ) ) ;
#6986=CARTESIAN_POINT ( 'NONE',  ( 7.771282357155271825, 9.000000000000000000, -3.443424244174282389 ) ) ;
#6994=LINE ( 'NONE', #5819, #9732 ) ;
#7004=ADVANCED_FACE ( 'NONE', ( #573 ), #7902, .T. ) ;
#7006=CARTESIAN_POINT ( 'NONE',  ( 7.110882674384088276, 9.000000000000000000, -3.538387050178523729 ) ) ;
#7010=ORIENTED_EDGE ( 'NONE', *, *, #11211, .F. ) ;
#7012=VERTEX_POINT ( 'NONE', #9098 ) ;
#7015=ORIENTED_EDGE ( 'NONE', *, *, #969, .T. ) ;
#7023=CARTESIAN_POINT ( 'NONE',  ( -0.8973464813148227526, 0.000000000000000000, -7.308217849399443189 ) ) ;
#7034=CARTESIAN_POINT ( 'NONE',  ( 3.007863545083557355, 0.000000000000000000, 7.350755164602351677 ) ) ;
#7045=LINE ( 'NONE', #12441, #1377 ) ;
#7064=EDGE_CURVE ( 'NONE', #5615, #6374, #12953, .T. ) ;
#7071=CIRCLE ( 'NONE', #7930, 6.750000000000000888 ) ;
#7074=CARTESIAN_POINT ( 'NONE',  ( 5.053288777954491273, 1.734723475976807094E-15, -4.475128213425755952 ) ) ;
#7082=CARTESIAN_POINT ( 'NONE',  ( 0.000000000000000000, 9.000000000000000000, 0.000000000000000000 ) ) ;
#7087=AXIS2_PLACEMENT_3D ( 'NONE', #1483, #5611, #8762 ) ;
#7099=ORIENTED_EDGE ( 'NONE', *, *, #6250, .T. ) ;
#7100=VECTOR ( 'NONE', #9586, 1000.000000000000000 ) ;
#7103=CARTESIAN_POINT ( 'NONE',  ( -3.533475733155565290, 9.000000000000000000, 7.730753471893975437 ) ) ;
#7104=VECTOR ( 'NONE', #12903, 1000.000000000000000 ) ;
#7115=ADVANCED_FACE ( 'NONE', ( #12433 ), #9167, .T. ) ;
#7122=CARTESIAN_POINT ( 'NONE',  ( -2.632142621505047408, 9.000000000000000000, -6.877144614729746586 ) ) ;
#7129=CARTESIAN_POINT ( 'NONE',  ( 3.818534268238711782, 9.000000000000000000, -5.566084444408534004 ) ) ;
#7132=CARTESIAN_POINT ( 'NONE',  ( 4.898587196589413075E-17, 0.000000000000000000, 0.4000000000000000222 ) ) ;
#7150=CARTESIAN_POINT ( 'NONE',  ( 0.000000000000000000, 0.000000000000000000, 9.250000000000000000 ) ) ;
#7151=CYLINDRICAL_SURFACE ( 'NONE', #3531, 9.250000000000000000 ) ;
#7153=AXIS2_PLACEMENT_3D ( 'NONE', #6837, #9865, #10009 ) ;
#7160=ADVANCED_FACE ( 'NONE', ( #6270 ), #8388, .T. ) ;
#7161=DIRECTION ( 'NONE',  ( -0.000000000000000000, -1.000000000000000000, -0.000000000000000000 ) ) ;
#7170=VERTEX_POINT ( 'NONE', #1882 ) ;
#7178=CARTESIAN_POINT ( 'NONE',  ( 2.620242232815953809, 9.000000000000000000, 6.881105251569436199 ) ) ;
#7179=CARTESIAN_POINT ( 'NONE',  ( 7.758214145541979967, 9.000000000000000000, 1.700281702449083054 ) ) ;
#7190=VERTEX_POINT ( 'NONE', #13579 ) ;
#7191=CARTESIAN_POINT ( 'NONE',  ( -4.174571361198896824, -1.694065894508600678E-18, 6.065330394303907191 ) ) ;
#7192=ORIENTED_EDGE ( 'NONE', *, *, #510, .T. ) ;
#7195=CARTESIAN_POINT ( 'NONE',  ( -5.496871281090180972, 0.000000000000000000, 4.899765193453235135 ) ) ;
#7198=DIRECTION ( 'NONE',  ( -0.000000000000000000, -1.000000000000000000, -0.000000000000000000 ) ) ;
#7203=CARTESIAN_POINT ( 'NONE',  ( -5.977417671213807182, 1.734723475976807094E-15, 3.135757960025121527 ) ) ;
#7206=ORIENTED_EDGE ( 'NONE', *, *, #5922, .T. ) ;
#7216=DIRECTION ( 'NONE',  ( 0.000000000000000000, 1.000000000000000000, -0.000000000000000000 ) ) ;
#7228=B_SPLINE_CURVE_WITH_KNOTS ( 'NONE', 3,
 ( #183, #3326, #11746, #6508 ),
 .UNSPECIFIED., .F., .F.,
 ( 4, 4 ),
 ( 0.1276832474596253097, 1.000000000000000000 ),
 .UNSPECIFIED. ) ;
#7238=VERTEX_POINT ( 'NONE', #10684 ) ;
#7248=EDGE_CURVE ( 'NONE', #7648, #1815, #11812, .T. ) ;
#7250=EDGE_CURVE ( 'NONE', #10192, #710, #5244, .T. ) ;
#7251=CARTESIAN_POINT ( 'NONE',  ( 6.554160776451332993, 9.000000000000000000, -1.614148852004323675 ) ) ;
#7256=CARTESIAN_POINT ( 'NONE',  ( 4.164551629694410728, 9.000000000000000000, -6.072874324029720050 ) ) ;
#7264=CARTESIAN_POINT ( 'NONE',  ( -7.144272221052618832, 9.000000000000000000, 1.784003156764502940 ) ) ;
#7281=B_SPLINE_CURVE_WITH_KNOTS ( 'NONE', 3,
 ( #12163, #10149, #12813, #11397 ),
 .UNSPECIFIED., .F., .F.,
 ( 4, 4 ),
 ( 0.1276832474596238665, 1.000000000000000000 ),
 .UNSPECIFIED. ) ;
#7288=CARTESIAN_POINT ( 'NONE',  ( -7.668956737359326148, 0.000000000000000000, -2.066866683227997825 ) ) ;
#7291=CARTESIAN_POINT ( 'NONE',  ( 6.554160776451332993, 9.000000000000000000, -1.614148852004323675 ) ) ;
#7298=ORIENTED_EDGE ( 'NONE', *, *, #1720, .T. ) ;
#7311=CARTESIAN_POINT ( 'NONE',  ( -2.481593227817850966, 9.000000000000000000, -8.129679886173169834 ) ) ;
#7317=CARTESIAN_POINT ( 'NONE',  ( 0.000000000000000000, 0.000000000000000000, 0.000000000000000000 ) ) ;
#7326=CARTESIAN_POINT ( 'NONE',  ( -7.780961115628988622, 9.000000000000000000, -3.421497350147985728 ) ) ;
#7327=CARTESIAN_POINT ( 'NONE',  ( -4.174571361198896824, 9.000000000000000000, 6.065330394303907191 ) ) ;
#7331=VERTEX_POINT ( 'NONE', #3368 ) ;
#7332=AXIS2_PLACEMENT_3D ( 'NONE', #7082, #13284, #3842 ) ;
#7339=EDGE_CURVE ( 'NONE', #3503, #7648, #2405, .T. ) ;
#7340=EDGE_CURVE ( 'NONE', #7331, #8551, #6636, .T. ) ;
#7345=EDGE_CURVE ( 'NONE', #10414, #12082, #12377, .T. ) ;
#7352=AXIS2_PLACEMENT_3D ( 'NONE', #9772, #7703, #11778 ) ;
#7353=VERTEX_POINT ( 'NONE', #10805 ) ;
#7370=CARTESIAN_POINT ( 'NONE',  ( 0.000000000000000000, 9.000000000000000000, 0.000000000000000000 ) ) ;
#7371=ORIENTED_EDGE ( 'NONE', *, *, #2172, .F. ) ;
#7381=CARTESIAN_POINT ( 'NONE',  ( -2.375523406013128724, 9.000000000000000000, 6.318179211409233886 ) ) ;
#7388=EDGE_LOOP ( 'NONE', ( #4682, #13303, #1792, #5408 ) ) ;
#7389=LINE ( 'NONE', #9515, #7100 ) ;
#7395=CARTESIAN_POINT ( 'NONE',  ( -6.749999880766614169, 9.000000000000000000, -0.001268720102703135150 ) ) ;
#7398=EDGE_CURVE ( 'NONE', #175, #6767, #11265, .T. ) ;
#7402=VERTEX_POINT ( 'NONE', #8792 ) ;
#7413=DIRECTION ( 'NONE',  ( 0.000000000000000000, -1.000000000000000000, 0.000000000000000000 ) ) ;
#7419=B_SPLINE_SURFACE_WITH_KNOTS ( 'NONE', 3, 1, ( 
 ( #13451, #4200 ),
 ( #8396, #3100 ),
 ( #12625, #3930 ),
 ( #7311, #2081 ) ),
 .UNSPECIFIED., .F., .F., .F.,
 ( 4, 4 ),
 ( 2, 2 ),
 ( 0.000000000000000000, 0.8724294488011762327 ),
 ( 0.000000000000000000, 1.000000000000000000 ),
 .UNSPECIFIED. ) ;
#7425=CARTESIAN_POINT ( 'NONE',  ( 7.248474140376192310, 9.000000000000000000, 4.439552076088041588 ) ) ;
#7441=DIRECTION ( 'NONE',  ( -0.000000000000000000, -1.000000000000000000, -0.000000000000000000 ) ) ;
#7449=ORIENTED_EDGE ( 'NONE', *, *, #11492, .F. ) ;
#7453=VERTEX_POINT ( 'NONE', #7705 ) ;
#7471=CARTESIAN_POINT ( 'NONE',  ( 0.000000000000000000, 9.000000000000000000, 0.000000000000000000 ) ) ;
#7478=ORIENTED_EDGE ( 'NONE', *, *, #3581, .F. ) ;
#7486=DIRECTION ( 'NONE',  ( -0.000000000000000000, -1.000000000000000000, -0.000000000000000000 ) ) ;
#7488=EDGE_CURVE ( 'NONE', #9824, #4801, #3562, .T. ) ;
#7494=ORIENTED_EDGE ( 'NONE', *, *, #9108, .F. ) ;
#7502=CARTESIAN_POINT ( 'NONE',  ( 0.000000000000000000, -3.000000000000000000, 0.000000000000000000 ) ) ;
#7509=ORIENTED_EDGE ( 'NONE', *, *, #12490, .F. ) ;
#7511=CARTESIAN_POINT ( 'NONE',  ( 7.363612555047485131, 9.000000000000000000, -0.02242701489043354146 ) ) ;
#7523=DIRECTION ( 'NONE',  ( -0.000000000000000000, -1.000000000000000000, -0.000000000000000000 ) ) ;
#7534=ORIENTED_EDGE ( 'NONE', *, *, #9266, .F. ) ;
#7536=AXIS2_PLACEMENT_3D ( 'NONE', #8600, #7713, #5442 ) ;
#7537=AXIS2_PLACEMENT_3D ( 'NONE', #10249, #945, #745 ) ;
#7539=FACE_OUTER_BOUND ( 'NONE', #3397, .T. ) ;
#7545=AXIS2_PLACEMENT_3D ( 'NONE', #9274, #10456, #1018 ) ;
#7546=CARTESIAN_POINT ( 'NONE',  ( 0.000000000000000000, 9.000000000000000000, 0.000000000000000000 ) ) ;
#7557=FACE_OUTER_BOUND ( 'NONE', #7388, .T. ) ;
#7561=DIRECTION ( 'NONE',  ( 0.000000000000000000, 0.000000000000000000, 1.000000000000000000 ) ) ;
#7574=VECTOR ( 'NONE', #3623, 1000.000000000000000 ) ;
#7581=LINE ( 'NONE', #3297, #9304 ) ;
#7593=ADVANCED_FACE ( 'NONE', ( #10184 ), #762, .T. ) ;
#7598=( GEOMETRIC_REPRESENTATION_CONTEXT ( 3 ) GLOBAL_UNCERTAINTY_ASSIGNED_CONTEXT ( ( #6962 ) ) GLOBAL_UNIT_ASSIGNED_CONTEXT ( ( #2357, #8883, #3446 ) ) REPRESENTATION_CONTEXT ( 'NONE', 'WORKASPACE' ) );
#7603=ORIENTED_EDGE ( 'NONE', *, *, #9036, .T. ) ;
#7611=EDGE_CURVE ( 'NONE', #4686, #7453, #6056, .T. ) ;
#7626=CARTESIAN_POINT ( 'NONE',  ( 3.818534268238711338, 0.000000000000000000, -5.566084444408533116 ) ) ;
#7635=ORIENTED_EDGE ( 'NONE', *, *, #609, .F. ) ;
#7645=ORIENTED_EDGE ( 'NONE', *, *, #7488, .F. ) ;
#7648=VERTEX_POINT ( 'NONE', #3535 ) ;
#7651=EDGE_LOOP ( 'NONE', ( #2132, #6466, #6126, #10555 ) ) ;
#7657=CARTESIAN_POINT ( 'NONE',  ( 0.000000000000000000, 9.000000000000000000, 0.000000000000000000 ) ) ;
#7658=DIRECTION ( 'NONE',  ( -0.000000000000000000, -1.000000000000000000, -0.000000000000000000 ) ) ;
#7666=ORIENTED_EDGE ( 'NONE', *, *, #4327, .T. ) ;
#7667=CARTESIAN_POINT ( 'NONE',  ( 7.151505841916629080, 0.000000000000000000, 1.752496229622501511 ) ) ;
#7672=CARTESIAN_POINT ( 'NONE',  ( 1.132798289211301698E-15, -3.000000000000000000, -9.250000000000000000 ) ) ;
#7681=ORIENTED_EDGE ( 'NONE', *, *, #720, .T. ) ;
#7685=DIRECTION ( 'NONE',  ( -0.000000000000000000, -1.000000000000000000, -0.000000000000000000 ) ) ;
#7687=CIRCLE ( 'NONE', #10102, 8.500000000000000000 ) ;
#7688=CARTESIAN_POINT ( 'NONE',  ( 5.985774866078161338, 9.000000000000000000, 3.119775513178307147 ) ) ;
#7694=EDGE_LOOP ( 'NONE', ( #10753, #2675, #3517, #8488, #9063, #9713, #4101, #13191, #3175, #3954, #3841, #12956, #11787, #12647, #6231, #1205, #4702, #13522, #8815, #3285, #11619, #2017, #282, #1604, #11591, #12422, #6975, #5094, #10457, #6850, #11554, #4628, #4319, #12523, #5990, #188, #11795, #339, #8719, #12486, #12969, #5822, #13525, #2480, #9981, #4944, #12076, #5289, #11856, #4836, #12016, #2608, #765 ) ) ;
#7702=EDGE_CURVE ( 'NONE', #11016, #4379, #9930, .T. ) ;
#7703=DIRECTION ( 'NONE',  ( 0.000000000000000000, 1.000000000000000000, -0.000000000000000000 ) ) ;
#7705=CARTESIAN_POINT ( 'NONE',  ( 0.4639228963249704130, 0.000000000000000000, 8.487330295579726069 ) ) ;
#7708=VERTEX_POINT ( 'NONE', #187 ) ;
#7709=CARTESIAN_POINT ( 'NONE',  ( 8.481367827640703183, 9.000000000000000000, 0.5624942419805127880 ) ) ;
#7710=EDGE_CURVE ( 'NONE', #7190, #5839, #934, .T. ) ;
#7713=DIRECTION ( 'NONE',  ( -0.000000000000000000, -1.000000000000000000, -0.000000000000000000 ) ) ;
#7728=VERTEX_POINT ( 'NONE', #6714 ) ;
#7745=B_SPLINE_SURFACE_WITH_KNOTS ( 'NONE', 3, 1, ( 
 ( #2224, #9797 ),
 ( #8691, #11866 ),
 ( #373, #4564 ),
 ( #6427, #10639 ) ),
 .UNSPECIFIED., .F., .F., .F.,
 ( 4, 4 ),
 ( 2, 2 ),
 ( 0.1276832474596270861, 1.000000000000000000 ),
 ( 0.000000000000000000, 1.000000000000000000 ),
 .UNSPECIFIED. ) ;
#7753=CARTESIAN_POINT ( 'NONE',  ( 1.132798289211301698E-15, 0.000000000000000000, -9.250000000000000000 ) ) ;
#7755=EDGE_CURVE ( 'NONE', #7331, #3742, #10645, .T. ) ;
#7757=CARTESIAN_POINT ( 'NONE',  ( 4.652003457867571967, 0.000000000000000000, -6.437678087145717321 ) ) ;
#7758=DIRECTION ( 'NONE',  ( -0.000000000000000000, -1.000000000000000000, -0.000000000000000000 ) ) ;
#7769=EDGE_CURVE ( 'NONE', #5694, #912, #6994, .T. ) ;
#7771=FACE_OUTER_BOUND ( 'NONE', #8515, .T. ) ;
#7772=ADVANCED_FACE ( 'NONE', ( #9186 ), #10980, .T. ) ;
#7783=FACE_OUTER_BOUND ( 'NONE', #11786, .T. ) ;
#7792=CARTESIAN_POINT ( 'NONE',  ( -8.100301009650792139, 9.000000000000000000, -2.575873357339267589 ) ) ;
#7795=VERTEX_POINT ( 'NONE', #3883 ) ;
#7807=FACE_OUTER_BOUND ( 'NONE', #56, .T. ) ;
#7816=DIRECTION ( 'NONE',  ( 0.000000000000000000, 1.000000000000000000, -0.000000000000000000 ) ) ;
#7824=LINE ( 'NONE', #1565, #9103 ) ;
#7830=CARTESIAN_POINT ( 'NONE',  ( 1.132798289211301698E-15, -3.000000000000000000, -9.250000000000000000 ) ) ;
#7850=CARTESIAN_POINT ( 'NONE',  ( 0.000000000000000000, 9.000000000000000000, 0.000000000000000000 ) ) ;
#7852=CARTESIAN_POINT ( 'NONE',  ( -5.526615004551211463, 0.000000000000000000, -4.866191470063547797 ) ) ;
#7858=B_SPLINE_SURFACE_WITH_KNOTS ( 'NONE', 3, 1, ( 
 ( #6638, #10845 ),
 ( #1212, #3606 ),
 ( #12917, #13049 ),
 ( #5402, #11748 ) ),
 .UNSPECIFIED., .F., .F., .F.,
 ( 4, 4 ),
 ( 2, 2 ),
 ( 0.1276832474596284739, 1.000000000000000000 ),
 ( 0.000000000000000000, 1.000000000000000000 ),
 .UNSPECIFIED. ) ;
#7862=CARTESIAN_POINT ( 'NONE',  ( 0.000000000000000000, 0.000000000000000000, 0.000000000000000000 ) ) ;
#7870=ADVANCED_FACE ( 'NONE', ( #4218, #9401 ), #114, .T. ) ;
#7871=CARTESIAN_POINT ( 'NONE',  ( -4.679611352264966051, -1.694065894508600678E-18, -6.417326716594978997 ) ) ;
#7875=CARTESIAN_POINT ( 'NONE',  ( -6.749999880766614169, 9.000000000000000000, -0.001268720102703135150 ) ) ;
#7876=ORIENTED_EDGE ( 'NONE', *, *, #6674, .F. ) ;
#7878=ORIENTED_EDGE ( 'NONE', *, *, #2374, .F. ) ;
#7883=CARTESIAN_POINT ( 'NONE',  ( 5.504794476853524188, 9.000000000000000000, -4.890042597913815570 ) ) ;
#7890=DIRECTION ( 'NONE',  ( 0.000000000000000000, 0.000000000000000000, -1.000000000000000000 ) ) ;
#7897=CARTESIAN_POINT ( 'NONE',  ( 6.554160776451332104, 0.000000000000000000, -1.614148852004323231 ) ) ;
#7898=CARTESIAN_POINT ( 'NONE',  ( -5.496871281090180972, 9.000000000000000000, 4.899765193453235135 ) ) ;
#7902=B_SPLINE_SURFACE_WITH_KNOTS ( 'NONE', 3, 1, ( 
 ( #4622, #3718 ),
 ( #12217, #703 ),
 ( #8954, #2496 ),
 ( #11027, #4696 ) ),
 .UNSPECIFIED., .F., .F., .F.,
 ( 4, 4 ),
 ( 2, 2 ),
 ( 0.000000000000000000, 0.8724294488011758997 ),
 ( 0.000000000000000000, 1.000000000000000000 ),
 .UNSPECIFIED. ) ;
#7910=VERTEX_POINT ( 'NONE', #2997 ) ;
#7920=EDGE_CURVE ( 'NONE', #10584, #8551, #9655, .T. ) ;
#7922=EDGE_CURVE ( 'NONE', #5839, #11792, #12022, .T. ) ;
#7930=AXIS2_PLACEMENT_3D ( 'NONE', #1446, #2603, #11081 ) ;
#7931=ORIENTED_EDGE ( 'NONE', *, *, #8235, .T. ) ;
#7937=CARTESIAN_POINT ( 'NONE',  ( 6.509732753943064054, 0.000000000000000000, -3.441899519755141412 ) ) ;
#7948=ORIENTED_EDGE ( 'NONE', *, *, #413, .F. ) ;
#7955=ADVANCED_FACE ( 'NONE', ( #1062 ), #39, .T. ) ;
#7960=CIRCLE ( 'NONE', #6419, 8.500000000000000000 ) ;
#7962=AXIS2_PLACEMENT_3D ( 'NONE', #13364, #7413, #10515 ) ;
#7964=FACE_OUTER_BOUND ( 'NONE', #13208, .T. ) ;
#7979=CARTESIAN_POINT ( 'NONE',  ( -1.161309641800940540, 0.000000000000000000, -7.856984441350959969 ) ) ;
#8011=CARTESIAN_POINT ( 'NONE',  ( 0.000000000000000000, 9.000000000000000000, 0.000000000000000000 ) ) ;
#8023=ORIENTED_EDGE ( 'NONE', *, *, #535, .T. ) ;
#8031=CARTESIAN_POINT ( 'NONE',  ( 5.280889752749253319, 0.000000000000000000, -6.660495733750448899 ) ) ;
#8054=FACE_OUTER_BOUND ( 'NONE', #5509, .T. ) ;
#8055=EDGE_CURVE ( 'NONE', #12363, #11178, #3235, .T. ) ;
#8062=B_SPLINE_CURVE_WITH_KNOTS ( 'NONE', 3,
 ( #11325, #918, #5190, #10142 ),
 .UNSPECIFIED., .F., .F.,
 ( 4, 4 ),
 ( 0.1276832474596304168, 1.000000000000000000 ),
 .UNSPECIFIED. ) ;
#8065=ORIENTED_EDGE ( 'NONE', *, *, #7488, .T. ) ;
#8077=CARTESIAN_POINT ( 'NONE',  ( -7.780961115628980629, 9.000000000000000000, -3.421497350147988392 ) ) ;
#8079=FACE_OUTER_BOUND ( 'NONE', #1776, .T. ) ;
#8080=( NAMED_UNIT ( * ) SI_UNIT ( $, .STERADIAN. ) SOLID_ANGLE_UNIT ( ) );
#8081=CARTESIAN_POINT ( 'NONE',  ( 7.248474140376191421, 0.000000000000000000, 4.439552076088042476 ) ) ;
#8087=CARTESIAN_POINT ( 'NONE',  ( 1.580708947611199511, 0.000000000000000000, -8.351727918397596540 ) ) ;
#8107=CARTESIAN_POINT ( 'NONE',  ( 8.481367827640703183, 0.000000000000000000, 0.5624942419805130100 ) ) ;
#8109=ORIENTED_EDGE ( 'NONE', *, *, #5146, .F. ) ;
#8114=DIRECTION ( 'NONE',  ( 0.000000000000000000, 0.000000000000000000, -1.000000000000000000 ) ) ;
#8125=ADVANCED_FACE ( 'NONE', ( #4499 ), #7745, .T. ) ;
#8129=CARTESIAN_POINT ( 'NONE',  ( -2.590203375110137873, 9.000000000000000000, 6.893050072893555758 ) ) ;
#8131=CARTESIAN_POINT ( 'NONE',  ( 0.7944557581062193785, 9.000000000000000000, -6.703084368289860429 ) ) ;
#8134=VERTEX_POINT ( 'NONE', #12769 ) ;
#8139=EDGE_LOOP ( 'NONE', ( #5560, #11842, #6977, #8765 ) ) ;
#8146=CARTESIAN_POINT ( 'NONE',  ( 5.053288777954491273, 1.734723475976807094E-15, -4.475128213425755952 ) ) ;
#8167=CARTESIAN_POINT ( 'NONE',  ( 7.363612555047485131, 0.000000000000000000, -0.02242701489043354146 ) ) ;
#8173=FACE_OUTER_BOUND ( 'NONE', #11129, .T. ) ;
#8178=CARTESIAN_POINT ( 'NONE',  ( -5.039625798601655937, 0.000000000000000000, 4.490509081392511703 ) ) ;
#8185=UNCERTAINTY_MEASURE_WITH_UNIT (LENGTH_MEASURE( 1.000000000000000082E-05 ), #1954, 'distance_accuracy_value', 'NONE');
#8187=ORIENTED_EDGE ( 'NONE', *, *, #4597, .F. ) ;
#8188=CARTESIAN_POINT ( 'NONE',  ( 0.4639228963249696913, 9.000000000000000000, 8.487330295579727846 ) ) ;
#8206=CARTESIAN_POINT ( 'NONE',  ( 7.771282357155270937, 9.000000000000000000, -3.443424244174282833 ) ) ;
#8226=VERTEX_POINT ( 'NONE', #5798 ) ;
#8235=EDGE_CURVE ( 'NONE', #2261, #3498, #9946, .T. ) ;
#8248=CIRCLE ( 'NONE', #4078, 6.749999999999999112 ) ;
#8250=DIRECTION ( 'NONE',  ( 0.000000000000000000, 0.000000000000000000, 1.000000000000000000 ) ) ;
#8256=CARTESIAN_POINT ( 'NONE',  ( 5.517918333394296049, 0.000000000000000000, 4.875228826198821253 ) ) ;
#8257=EDGE_CURVE ( 'NONE', #2790, #76, #2407, .T. ) ;
#8261=CARTESIAN_POINT ( 'NONE',  ( 0.000000000000000000, 0.000000000000000000, 0.000000000000000000 ) ) ;
#8265=EDGE_CURVE ( 'NONE', #710, #3254, #706, .T. ) ;
#8274=EDGE_CURVE ( 'NONE', #7331, #11192, #4773, .T. ) ;
#8278=VERTEX_POINT ( 'NONE', #2011 ) ;
#8285=CARTESIAN_POINT ( 'NONE',  ( -7.668956737359326148, 0.000000000000000000, -2.066866683227997825 ) ) ;
#8287=CARTESIAN_POINT ( 'NONE',  ( 6.079397157347990799, -1.694065894508600678E-18, 5.110946565852551693 ) ) ;
#8303=ORIENTED_EDGE ( 'NONE', *, *, #8959, .F. ) ;
#8304=CARTESIAN_POINT ( 'NONE',  ( -1.604252589105048976, 0.000000000000000000, -8.347237484961699039 ) ) ;
#8305=CARTESIAN_POINT ( 'NONE',  ( 3.850308450823737516, 9.000000000000000000, 5.544152309732777617 ) ) ;
#8310=PRODUCT_CONTEXT ( 'NONE', #4935, 'mechanical' ) ;
#8314=CARTESIAN_POINT ( 'NONE',  ( -7.780961115628980629, 0.000000000000000000, -3.421497350147988392 ) ) ;
#8318=CARTESIAN_POINT ( 'NONE',  ( 5.967832595844252630, 0.000000000000000000, -3.153961652902406154 ) ) ;
#8325=DIRECTION ( 'NONE',  ( -0.000000000000000000, -1.000000000000000000, -0.000000000000000000 ) ) ;
#8331=B_SPLINE_CURVE_WITH_KNOTS ( 'NONE', 3,
 ( #3652, #7852, #633, #1672 ),
 .UNSPECIFIED., .F., .F.,
 ( 4, 4 ),
 ( 0.000000000000000000, 0.8724294488011758997 ),
 .UNSPECIFIED. ) ;
#8336=DIRECTION ( 'NONE',  ( 0.000000000000000000, 0.000000000000000000, -1.000000000000000000 ) ) ;
#8352=EDGE_CURVE ( 'NONE', #12329, #5918, #11301, .T. ) ;
#8354=VERTEX_POINT ( 'NONE', #910 ) ;
#8367=DIRECTION ( 'NONE',  ( 0.000000000000000000, 0.000000000000000000, -1.000000000000000000 ) ) ;
#8376=SHAPE_REPRESENTATION ( 'base-gear', ( #10007 ), #6493 ) ;
#8383=DIRECTION ( 'NONE',  ( 0.000000000000000000, 0.000000000000000000, 1.000000000000000000 ) ) ;
#8387=CARTESIAN_POINT ( 'NONE',  ( -7.235926821844434365, 9.000000000000000000, 4.459973433655444630 ) ) ;
#8388=B_SPLINE_SURFACE_WITH_KNOTS ( 'NONE', 3, 1, ( 
 ( #8131, #11239 ),
 ( #5237, #4135 ),
 ( #3034, #10210 ),
 ( #1808, #2974 ) ),
 .UNSPECIFIED., .F., .F., .F.,
 ( 4, 4 ),
 ( 2, 2 ),
 ( 0.000000000000000000, 0.8724294488011757887 ),
 ( 0.000000000000000000, 1.000000000000000000 ),
 .UNSPECIFIED. ) ;
#8396=CARTESIAN_POINT ( 'NONE',  ( -2.632142621505047408, 9.000000000000000000, -6.877144614729746586 ) ) ;
#8398=AXIS2_PLACEMENT_3D ( 'NONE', #1581, #13088, #2548 ) ;
#8413=ADVANCED_FACE ( 'NONE', ( #12557 ), #7419, .T. ) ;
#8427=AXIS2_PLACEMENT_3D ( 'NONE', #6520, #6651, #11760 ) ;
#8434=ORIENTED_EDGE ( 'NONE', *, *, #279, .F. ) ;
#8439=CIRCLE ( 'NONE', #529, 8.500000000000000000 ) ;
#8443=CARTESIAN_POINT ( 'NONE',  ( -4.679611352264966051, 9.000000000000000000, -6.417326716594978997 ) ) ;
#8448=EDGE_CURVE ( 'NONE', #13005, #12082, #6334, .T. ) ;
#8463=EDGE_CURVE ( 'NONE', #12082, #3918, #5375, .T. ) ;
#8466=DIRECTION ( 'NONE',  ( 0.000000000000000000, -0.000000000000000000, -1.000000000000000000 ) ) ;
#8470=CARTESIAN_POINT ( 'NONE',  ( -8.369528376005813897, 9.000000000000000000, 1.483574994138650460 ) ) ;
#8488=ORIENTED_EDGE ( 'NONE', *, *, #11734, .F. ) ;
#8501=CARTESIAN_POINT ( 'NONE',  ( 4.355042381134428098, 9.000000000000000000, 7.299562031966232212 ) ) ;
#8509=EDGE_CURVE ( 'NONE', #7795, #8800, #7581, .T. ) ;
#8515=EDGE_LOOP ( 'NONE', ( #328, #7494, #5347, #7298 ) ) ;
#8516=ORIENTED_EDGE ( 'NONE', *, *, #10649, .F. ) ;
#8517=EDGE_LOOP ( 'NONE', ( #12662, #12696, #2571, #893 ) ) ;
#8521=CARTESIAN_POINT ( 'NONE',  ( 0.000000000000000000, 9.000000000000000000, 0.000000000000000000 ) ) ;
#8534=ORIENTED_EDGE ( 'NONE', *, *, #11123, .F. ) ;
#8551=VERTEX_POINT ( 'NONE', #8470 ) ;
#8557=CARTESIAN_POINT ( 'NONE',  ( 5.958322434183388694, 9.000000000000000000, -6.062045345451230638 ) ) ;
#8565=ORIENTED_EDGE ( 'NONE', *, *, #12589, .T. ) ;
#8577=ADVANCED_FACE ( 'NONE', ( #3642 ), #12276, .T. ) ;
#8580=VERTEX_POINT ( 'NONE', #558 ) ;
#8586=ORIENTED_EDGE ( 'NONE', *, *, #427, .T. ) ;
#8587=FACE_OUTER_BOUND ( 'NONE', #1949, .T. ) ;
#8600=CARTESIAN_POINT ( 'NONE',  ( 0.000000000000000000, 9.000000000000000000, 0.000000000000000000 ) ) ;
#8621=EDGE_LOOP ( 'NONE', ( #2738, #7645 ) ) ;
#8626=CARTESIAN_POINT ( 'NONE',  ( 0.000000000000000000, 0.000000000000000000, 0.000000000000000000 ) ) ;
#8631=DIRECTION ( 'NONE',  ( 0.000000000000000000, 1.000000000000000000, -0.000000000000000000 ) ) ;
#8644=CARTESIAN_POINT ( 'NONE',  ( 7.771282357155271825, 0.000000000000000000, -3.443424244174282389 ) ) ;
#8646=CYLINDRICAL_SURFACE ( 'NONE', #1984, 0.4000000000000000222 ) ;
#8650=FACE_OUTER_BOUND ( 'NONE', #4887, .T. ) ;
#8651=AXIS2_PLACEMENT_3D ( 'NONE', #2899, #4071, #12431 ) ;
#8655=VERTEX_POINT ( 'NONE', #2960 ) ;
#8658=EDGE_CURVE ( 'NONE', #1248, #7910, #2491, .T. ) ;
#8660=CIRCLE ( 'NONE', #4051, 6.749999999999999112 ) ;
#8668=ORIENTED_EDGE ( 'NONE', *, *, #7710, .T. ) ;
#8690=ORIENTED_EDGE ( 'NONE', *, *, #4470, .F. ) ;
#8691=CARTESIAN_POINT ( 'NONE',  ( 5.806472362263156661, 9.000000000000000000, -5.419014975255640465 ) ) ;
#8709=ADVANCED_FACE ( 'NONE', ( #6064 ), #5771, .T. ) ;
#8717=CARTESIAN_POINT ( 'NONE',  ( 0.000000000000000000, 0.000000000000000000, 0.000000000000000000 ) ) ;
#8719=ORIENTED_EDGE ( 'NONE', *, *, #2320, .T. ) ;
#8720=ORIENTED_EDGE ( 'NONE', *, *, #2320, .F. ) ;
#8729=CARTESIAN_POINT ( 'NONE',  ( 8.093005444143644311, 9.000000000000000000, -2.598704077239528676 ) ) ;
#8747=CARTESIAN_POINT ( 'NONE',  ( -0.8148820470561124463, 0.000000000000000000, 6.700631854488474204 ) ) ;
#8757=LINE ( 'NONE', #12152, #11911 ) ;
#8762=DIRECTION ( 'NONE',  ( 0.000000000000000000, 0.000000000000000000, 1.000000000000000000 ) ) ;
#8765=ORIENTED_EDGE ( 'NONE', *, *, #2532, .F. ) ;
#8775=DIRECTION ( 'NONE',  ( 0.000000000000000000, 0.000000000000000000, 1.000000000000000000 ) ) ;
#8790=CARTESIAN_POINT ( 'NONE',  ( 7.771282357155271825, 0.000000000000000000, -3.443424244174282389 ) ) ;
#8792=CARTESIAN_POINT ( 'NONE',  ( 1.580708947611199511, 9.000000000000000000, -8.351727918397596540 ) ) ;
#8797=ORIENTED_EDGE ( 'NONE', *, *, #8257, .T. ) ;
#8800=VERTEX_POINT ( 'NONE', #2252 ) ;
#8801=VECTOR ( 'NONE', #5740, 1000.000000000000000 ) ;
#8806=ADVANCED_FACE ( 'NONE', ( #8650 ), #2393, .T. ) ;
#8815=ORIENTED_EDGE ( 'NONE', *, *, #11663, .T. ) ;
#8833=AXIS2_PLACEMENT_3D ( 'NONE', #718, #2842, #1823 ) ;
#8834=VECTOR ( 'NONE', #13541, 1000.000000000000000 ) ;
#8839=DIRECTION ( 'NONE',  ( 0.000000000000000000, 0.000000000000000000, 1.000000000000000000 ) ) ;
#8841=CYLINDRICAL_SURFACE ( 'NONE', #504, 8.500000000000000000 ) ;
#8844=LINE ( 'NONE', #258, #5727 ) ;
#8862=CARTESIAN_POINT ( 'NONE',  ( 8.093005444143644311, 0.000000000000000000, -2.598704077239528676 ) ) ;
#8865=CARTESIAN_POINT ( 'NONE',  ( -7.780961115628980629, 9.000000000000000000, -3.421497350147988392 ) ) ;
#8873=ORIENTED_EDGE ( 'NONE', *, *, #11140, .F. ) ;
#8875=LINE ( 'NONE', #9783, #12608 ) ;
#8876=VERTEX_POINT ( 'NONE', #11899 ) ;
#8878=VECTOR ( 'NONE', #6525, 1000.000000000000000 ) ;
#8883=( NAMED_UNIT ( * ) PLANE_ANGLE_UNIT ( ) SI_UNIT ( $, .RADIAN. ) );
#8894=ORIENTED_EDGE ( 'NONE', *, *, #1522, .T. ) ;
#8908=DIRECTION ( 'NONE',  ( -0.000000000000000000, -1.000000000000000000, -0.000000000000000000 ) ) ;
#8920=CARTESIAN_POINT ( 'NONE',  ( 5.806472362263156661, 9.000000000000000000, -5.419014975255640465 ) ) ;
#8922=DIRECTION ( 'NONE',  ( 0.000000000000000000, 0.000000000000000000, 1.000000000000000000 ) ) ;
#8925=ADVANCED_FACE ( 'NONE', ( #7964 ), #5897, .T. ) ;
#8929=ADVANCED_FACE ( 'NONE', ( #6862 ), #10035, .T. ) ;
#8935=CARTESIAN_POINT ( 'NONE',  ( 7.146769547044127258, 0.000000000000000000, -1.771712133291270863 ) ) ;
#8936=CARTESIAN_POINT ( 'NONE',  ( -1.604252589105048976, 0.000000000000000000, -8.347237484961699039 ) ) ;
#8938=CARTESIAN_POINT ( 'NONE',  ( 7.110882674384088276, 0.000000000000000000, -3.538387050178523729 ) ) ;
#8945=VERTEX_POINT ( 'NONE', #2594 ) ;
#8954=CARTESIAN_POINT ( 'NONE',  ( -5.830003112347290184, 9.000000000000000000, -5.394061460138155795 ) ) ;
#8957=CARTESIAN_POINT ( 'NONE',  ( -8.479748006907131597, 9.000000000000000000, 0.5864074857593127854 ) ) ;
#8959=EDGE_CURVE ( 'NONE', #2737, #11339, #965, .T. ) ;
#8970=CARTESIAN_POINT ( 'NONE',  ( 3.850308450823737516, 0.000000000000000000, 5.544152309732777617 ) ) ;
#8971=DIRECTION ( 'NONE',  ( 0.000000000000000000, 0.000000000000000000, -1.000000000000000000 ) ) ;
#8975=ORIENTED_EDGE ( 'NONE', *, *, #10785, .T. ) ;
#8976=VERTEX_POINT ( 'NONE', #12324 ) ;
#9015=CYLINDRICAL_SURFACE ( 'NONE', #1379, 0.4000000000000000222 ) ;
#9021=CARTESIAN_POINT ( 'NONE',  ( -0.4399887592034530392, 0.000000000000000000, 8.488604708182295511 ) ) ;
#9024=DIRECTION ( 'NONE',  ( 0.000000000000000000, 1.000000000000000000, -0.000000000000000000 ) ) ;
#9028=CARTESIAN_POINT ( 'NONE',  ( -2.411622991978541464, 9.000000000000000000, -6.304488444319688689 ) ) ;
#9032=LINE ( 'NONE', #2506, #764 ) ;
#9036=EDGE_CURVE ( 'NONE', #5615, #7453, #13286, .T. ) ;
#9045=B_SPLINE_CURVE_WITH_KNOTS ( 'NONE', 3,
 ( #8314, #4055, #9287, #6062 ),
 .UNSPECIFIED., .F., .F.,
 ( 4, 4 ),
 ( 0.1276832474596248101, 1.000000000000000000 ),
 .UNSPECIFIED. ) ;
#9050=B_SPLINE_CURVE_WITH_KNOTS ( 'NONE', 3,
 ( #12038, #10862, #9820, #1429 ),
 .UNSPECIFIED., .F., .F.,
 ( 4, 4 ),
 ( 0.000000000000000000, 0.8724294488011757887 ),
 .UNSPECIFIED. ) ;
#9056=CARTESIAN_POINT ( 'NONE',  ( 6.509732753943064054, 9.000000000000000000, -3.441899519755141412 ) ) ;
#9057=CARTESIAN_POINT ( 'NONE',  ( 7.771282357155270937, 9.000000000000000000, -3.443424244174282833 ) ) ;
#9063=ORIENTED_EDGE ( 'NONE', *, *, #10527, .T. ) ;
#9091=AXIS2_PLACEMENT_3D ( 'NONE', #10024, #7816, #3678 ) ;
#9094=CARTESIAN_POINT ( 'NONE',  ( -6.934601996837493232, -1.694065894508600678E-18, 3.871968458191308748 ) ) ;
#9095=B_SPLINE_SURFACE_WITH_KNOTS ( 'NONE', 3, 1, ( 
 ( #11457, #1960 ),
 ( #9453, #4152 ),
 ( #7327, #13397 ),
 ( #6152, #36 ) ),
 .UNSPECIFIED., .F., .F., .F.,
 ( 4, 4 ),
 ( 2, 2 ),
 ( 0.1276832474596244493, 1.000000000000000000 ),
 ( 0.000000000000000000, 1.000000000000000000 ),
 .UNSPECIFIED. ) ;
#9096=CARTESIAN_POINT ( 'NONE',  ( -2.375523406013125616, 0.000000000000000000, 6.318179211409232998 ) ) ;
#9097=CARTESIAN_POINT ( 'NONE',  ( -7.155006492985575228, 9.000000000000000000, -1.740452503570284915 ) ) ;
#9098=CARTESIAN_POINT ( 'NONE',  ( -7.235926821844430812, 0.000000000000000000, 4.459973433655439301 ) ) ;
#9103=VECTOR ( 'NONE', #4737, 1000.000000000000000 ) ;
#9106=CARTESIAN_POINT ( 'NONE',  ( 6.553553527263006551, 1.734723475976807094E-15, 1.616612558808879774 ) ) ;
#9108=EDGE_CURVE ( 'NONE', #933, #4948, #1599, .T. ) ;
#9109=ORIENTED_EDGE ( 'NONE', *, *, #5186, .F. ) ;
#9122=VECTOR ( 'NONE', #9847, 1000.000000000000000 ) ;
#9123=B_SPLINE_CURVE_WITH_KNOTS ( 'NONE', 3,
 ( #7129, #7256, #11327, #4147 ),
 .UNSPECIFIED., .F., .F.,
 ( 4, 4 ),
 ( 0.000000000000000000, 0.8724294488011765658 ),
 .UNSPECIFIED. ) ;
#9147=ORIENTED_EDGE ( 'NONE', *, *, #8448, .T. ) ;
#9148=CARTESIAN_POINT ( 'NONE',  ( 0.000000000000000000, 0.000000000000000000, 0.000000000000000000 ) ) ;
#9154=CARTESIAN_POINT ( 'NONE',  ( -6.558450276537426404, 0.000000000000000000, -1.596630818375423866 ) ) ;
#9158=ORIENTED_EDGE ( 'NONE', *, *, #4091, .T. ) ;
#9159=ORIENTED_EDGE ( 'NONE', *, *, #11832, .F. ) ;
#9165=DIRECTION ( 'NONE',  ( -0.000000000000000000, -1.000000000000000000, -0.000000000000000000 ) ) ;
#9167=CYLINDRICAL_SURFACE ( 'NONE', #11923, 8.499999999999992895 ) ;
#9172=ORIENTED_EDGE ( 'NONE', *, *, #7, .F. ) ;
#9184=EDGE_CURVE ( 'NONE', #7012, #3254, #2467, .T. ) ;
#9186=FACE_OUTER_BOUND ( 'NONE', #3376, .T. ) ;
#9188=EDGE_CURVE ( 'NONE', #1159, #10417, #5334, .T. ) ;
#9189=EDGE_LOOP ( 'NONE', ( #12890, #8690, #12942, #768 ) ) ;
#9198=EDGE_CURVE ( 'NONE', #75, #3196, #6433, .T. ) ;
#9207=ORIENTED_EDGE ( 'NONE', *, *, #2374, .T. ) ;
#9211=FACE_OUTER_BOUND ( 'NONE', #8517, .T. ) ;
#9217=CARTESIAN_POINT ( 'NONE',  ( 6.079397157347990799, 0.000000000000000000, 5.110946565852551693 ) ) ;
#9223=B_SPLINE_CURVE_WITH_KNOTS ( 'NONE', 3,
 ( #12777, #1267, #6634, #1330 ),
 .UNSPECIFIED., .F., .F.,
 ( 4, 4 ),
 ( 0.1276832474596256706, 1.000000000000000000 ),
 .UNSPECIFIED. ) ;
#9226=CARTESIAN_POINT ( 'NONE',  ( 7.151505841916629080, 9.000000000000000000, 1.752496229622501511 ) ) ;
#9230=VECTOR ( 'NONE', #7523, 1000.000000000000000 ) ;
#9240=ADVANCED_FACE ( 'NONE', ( #4985 ), #10503, .T. ) ;
#9241=DIRECTION ( 'NONE',  ( 0.000000000000000000, 1.000000000000000000, -0.000000000000000000 ) ) ;
#9248=FACE_OUTER_BOUND ( 'NONE', #12245, .T. ) ;
#9252=VECTOR ( 'NONE', #3636, 1000.000000000000000 ) ;
#9266=EDGE_CURVE ( 'NONE', #7795, #12927, #9123, .T. ) ;
#9273=CARTESIAN_POINT ( 'NONE',  ( 0.000000000000000000, 9.000000000000000000, 0.000000000000000000 ) ) ;
#9274=CARTESIAN_POINT ( 'NONE',  ( 0.000000000000000000, 9.000000000000000000, 0.000000000000000000 ) ) ;
#9277=B_SPLINE_CURVE_WITH_KNOTS ( 'NONE', 3,
 ( #6811, #6964, #13223, #7103 ),
 .UNSPECIFIED., .F., .F.,
 ( 4, 4 ),
 ( 0.000000000000000000, 0.8724294488011768989 ),
 .UNSPECIFIED. ) ;
#9285=DIRECTION ( 'NONE',  ( 0.000000000000000000, 0.000000000000000000, 1.000000000000000000 ) ) ;
#9287=CARTESIAN_POINT ( 'NONE',  ( -6.524296280129988190, 0.000000000000000000, -3.413039245436654490 ) ) ;
#9289=CARTESIAN_POINT ( 'NONE',  ( 6.079397157347990799, 9.000000000000000000, 5.110946565852551693 ) ) ;
#9298=DIRECTION ( 'NONE',  ( 0.000000000000000000, 0.000000000000000000, 1.000000000000000000 ) ) ;
#9300=CARTESIAN_POINT ( 'NONE',  ( 8.373678438139048552, 9.000000000000000000, 1.459968977288628178 ) ) ;
#9303=CIRCLE ( 'NONE', #6444, 6.750000000000000888 ) ;
#9304=VECTOR ( 'NONE', #5501, 1000.000000000000000 ) ;
#9316=CIRCLE ( 'NONE', #4247, 6.750000000000000888 ) ;
#9322=CARTESIAN_POINT ( 'NONE',  ( 2.458659560121117416, 0.000000000000000000, -8.136645080586040635 ) ) ;
#9327=CARTESIAN_POINT ( 'NONE',  ( -0.8123631076467130452, 1.734723475976807094E-15, -6.700937709107178009 ) ) ;
#9330=ORIENTED_EDGE ( 'NONE', *, *, #10350, .F. ) ;
#9353=FACE_OUTER_BOUND ( 'NONE', #10853, .T. ) ;
#9355=CARTESIAN_POINT ( 'NONE',  ( -5.299649803506881085, 9.000000000000000000, -6.645578376649351249 ) ) ;
#9358=COLOUR_RGB ( '',0.7803921568627451011, 0.7607843137254901578, 0.7411764705882353255 ) ;
#9361=CARTESIAN_POINT ( 'NONE',  ( -8.100301009650792139, 9.000000000000000000, -2.575873357339267589 ) ) ;
#9377=CARTESIAN_POINT ( 'NONE',  ( -2.976187484161006314, 9.000000000000000000, 7.363908159724035229 ) ) ;
#9390=DIRECTION ( 'NONE',  ( -0.000000000000000000, -1.000000000000000000, -0.000000000000000000 ) ) ;
#9392=CARTESIAN_POINT ( 'NONE',  ( 2.394769219159762930, 9.000000000000000000, -6.310909632292713844 ) ) ;
#9401=FACE_BOUND ( 'NONE', #13419, .T. ) ;
#9424=ORIENTED_EDGE ( 'NONE', *, *, #2232, .F. ) ;
#9425=ORIENTED_EDGE ( 'NONE', *, *, #7611, .F. ) ;
#9431=DIRECTION ( 'NONE',  ( -0.000000000000000000, -1.000000000000000000, -0.000000000000000000 ) ) ;
#9433=DIRECTION ( 'NONE',  ( 0.000000000000000000, 0.000000000000000000, 1.000000000000000000 ) ) ;
#9444=EDGE_CURVE ( 'NONE', #11926, #6767, #297, .T. ) ;
#9453=CARTESIAN_POINT ( 'NONE',  ( -4.340891659662447388, 9.000000000000000000, 6.651128039276029469 ) ) ;
#9459=VECTOR ( 'NONE', #7198, 1000.000000000000000 ) ;
#9464=VERTEX_POINT ( 'NONE', #10756 ) ;
#9469=CARTESIAN_POINT ( 'NONE',  ( 8.093005444143644311, 0.000000000000000000, -2.598704077239528232 ) ) ;
#9477=VECTOR ( 'NONE', #679, 1000.000000000000000 ) ;
#9481=CARTESIAN_POINT ( 'NONE',  ( 0.000000000000000000, 9.000000000000000000, -0.4000000000000000222 ) ) ;
#9483=FACE_OUTER_BOUND ( 'NONE', #8621, .T. ) ;
#9492=ORIENTED_EDGE ( 'NONE', *, *, #6836, .T. ) ;
#9497=CARTESIAN_POINT ( 'NONE',  ( -6.515098946627274401, 9.000000000000000000, 3.430563300314522390 ) ) ;
#9514=ORIENTED_EDGE ( 'NONE', *, *, #7922, .F. ) ;
#9515=CARTESIAN_POINT ( 'NONE',  ( 5.958322434183388694, 9.000000000000000000, -6.062045345451230638 ) ) ;
#9516=B_SPLINE_CURVE_WITH_KNOTS ( 'NONE', 3,
 ( #1750, #7195, #10347, #919 ),
 .UNSPECIFIED., .F., .F.,
 ( 4, 4 ),
 ( 0.000000000000000000, 0.8724294488011775650 ),
 .UNSPECIFIED. ) ;
#9527=B_SPLINE_SURFACE_WITH_KNOTS ( 'NONE', 3, 1, ( 
 ( #12995, #7626 ),
 ( #9882, #5683 ),
 ( #533, #7757 ),
 ( #11065, #10990 ) ),
 .UNSPECIFIED., .F., .F., .F.,
 ( 4, 4 ),
 ( 2, 2 ),
 ( 0.000000000000000000, 0.8724294488011765658 ),
 ( 0.000000000000000000, 1.000000000000000000 ),
 .UNSPECIFIED. ) ;
#9532=ADVANCED_FACE ( 'NONE', ( #5791 ), #9015, .F. ) ;
#9539=ORIENTED_EDGE ( 'NONE', *, *, #2733, .T. ) ;
#9541=EDGE_CURVE ( 'NONE', #7012, #6815, #12733, .T. ) ;
#9546=VECTOR ( 'NONE', #7441, 1000.000000000000000 ) ;
#9563=DIRECTION ( 'NONE',  ( -0.000000000000000000, -1.000000000000000000, -0.000000000000000000 ) ) ;
#9566=DIRECTION ( 'NONE',  ( 0.000000000000000000, 1.000000000000000000, -0.000000000000000000 ) ) ;
#9569=ORIENTED_EDGE ( 'NONE', *, *, #2793, .T. ) ;
#9573=DIRECTION ( 'NONE',  ( 0.000000000000000000, 0.000000000000000000, 1.000000000000000000 ) ) ;
#9577=CARTESIAN_POINT ( 'NONE',  ( -7.668956737359326148, 9.000000000000000000, -2.066866683227997825 ) ) ;
#9586=DIRECTION ( 'NONE',  ( -0.000000000000000000, -1.000000000000000000, -0.000000000000000000 ) ) ;
#9595=FACE_OUTER_BOUND ( 'NONE', #767, .T. ) ;
#9600=VERTEX_POINT ( 'NONE', #4893 ) ;
#9604=CARTESIAN_POINT ( 'NONE',  ( 8.373678438139048552, 0.000000000000000000, 1.459968977288628844 ) ) ;
#9608=CARTESIAN_POINT ( 'NONE',  ( -6.549210654805285969, 9.000000000000000000, 1.634117437329680067 ) ) ;
#9629=ORIENTED_EDGE ( 'NONE', *, *, #1522, .F. ) ;
#9637=FACE_OUTER_BOUND ( 'NONE', #12547, .T. ) ;
#9646=ORIENTED_EDGE ( 'NONE', *, *, #11804, .F. ) ;
#9647=DIRECTION ( 'NONE',  ( -0.000000000000000000, -1.000000000000000000, -0.000000000000000000 ) ) ;
#9655=B_SPLINE_CURVE_WITH_KNOTS ( 'NONE', 3,
 ( #11535, #7264, #929, #5124 ),
 .UNSPECIFIED., .F., .F.,
 ( 4, 4 ),
 ( 0.000000000000000000, 0.8724294488011786752 ),
 .UNSPECIFIED. ) ;
#9676=CARTESIAN_POINT ( 'NONE',  ( 4.355042381134428098, 0.000000000000000000, 7.299562031966232212 ) ) ;
#9679=LINE ( 'NONE', #3214, #6678 ) ;
#9694=EDGE_LOOP ( 'NONE', ( #13280, #3951, #10363, #10088 ) ) ;
#9698=EDGE_CURVE ( 'NONE', #10414, #1535, #11898, .T. ) ;
#9703=DIRECTION ( 'NONE',  ( 0.000000000000000000, 0.000000000000000000, 1.000000000000000000 ) ) ;
#9713=ORIENTED_EDGE ( 'NONE', *, *, #720, .F. ) ;
#9714=EDGE_LOOP ( 'NONE', ( #7603, #4594, #747, #13056 ) ) ;
#9715=DIRECTION ( 'NONE',  ( 0.000000000000000000, 1.000000000000000000, -0.000000000000000000 ) ) ;
#9722=CARTESIAN_POINT ( 'NONE',  ( -3.835481108877868195, 1.734723475976807094E-15, 5.554420281491219136 ) ) ;
#9732=VECTOR ( 'NONE', #11190, 1000.000000000000000 ) ;
#9742=ORIENTED_EDGE ( 'NONE', *, *, #7339, .F. ) ;
#9751=CARTESIAN_POINT ( 'NONE',  ( -2.375523406013128724, 9.000000000000000000, 6.318179211409233886 ) ) ;
#9760=ORIENTED_EDGE ( 'NONE', *, *, #6082, .F. ) ;
#9762=VERTEX_POINT ( 'NONE', #3924 ) ;
#9772=CARTESIAN_POINT ( 'NONE',  ( 0.000000000000000000, 0.000000000000000000, 0.000000000000000000 ) ) ;
#9774=CARTESIAN_POINT ( 'NONE',  ( 0.000000000000000000, 9.000000000000000000, 0.000000000000000000 ) ) ;
#9783=CARTESIAN_POINT ( 'NONE',  ( -2.411622991978541464, 9.000000000000000000, -6.304488444319688689 ) ) ;
#9793=CARTESIAN_POINT ( 'NONE',  ( -0.8148820470561124463, 9.000000000000000000, 6.700631854488474204 ) ) ;
#9794=B_SPLINE_CURVE_WITH_KNOTS ( 'NONE', 3,
 ( #13356, #2049, #12326, #12473 ),
 .UNSPECIFIED., .F., .F.,
 ( 4, 4 ),
 ( 0.000000000000000000, 0.8724294488011786752 ),
 .UNSPECIFIED. ) ;
#9797=CARTESIAN_POINT ( 'NONE',  ( 5.958322434183389582, 0.000000000000000000, -6.062045345451230638 ) ) ;
#9798=EDGE_CURVE ( 'NONE', #13005, #8655, #9303, .T. ) ;
#9799=EDGE_LOOP ( 'NONE', ( #209, #9742, #6614, #6853 ) ) ;
#9804=DIRECTION ( 'NONE',  ( 0.000000000000000000, 1.000000000000000000, -0.000000000000000000 ) ) ;
#9806=ADVANCED_FACE ( 'NONE', ( #5751 ), #8841, .T. ) ;
#9808=CARTESIAN_POINT ( 'NONE',  ( 7.940744365623959133, 9.000000000000000000, 0.1715058177969961128 ) ) ;
#9815=DIRECTION ( 'NONE',  ( -0.000000000000000000, -1.000000000000000000, -0.000000000000000000 ) ) ;
#9820=CARTESIAN_POINT ( 'NONE',  ( 1.127406311874972422, 0.000000000000000000, -7.862174656777307646 ) ) ;
#9824=VERTEX_POINT ( 'NONE', #7753 ) ;
#9846=EDGE_LOOP ( 'NONE', ( #11999, #100, #11073, #6032 ) ) ;
#9847=DIRECTION ( 'NONE',  ( -0.000000000000000000, -1.000000000000000000, -0.000000000000000000 ) ) ;
#9848=SURFACE_STYLE_USAGE ( .BOTH. , #12830 ) ;
#9862=ORIENTED_EDGE ( 'NONE', *, *, #11034, .T. ) ;
#9865=DIRECTION ( 'NONE',  ( 0.000000000000000000, 1.000000000000000000, -0.000000000000000000 ) ) ;
#9873=VERTEX_POINT ( 'NONE', #2136 ) ;
#9880=B_SPLINE_CURVE_WITH_KNOTS ( 'NONE', 3,
 ( #1123, #2992, #6221, #6094 ),
 .UNSPECIFIED., .F., .F.,
 ( 4, 4 ),
 ( 0.000000000000000000, 0.8724294488011765658 ),
 .UNSPECIFIED. ) ;
#9882=CARTESIAN_POINT ( 'NONE',  ( 4.164551629694410728, 9.000000000000000000, -6.072874324029720050 ) ) ;
#9889=ORIENTED_EDGE ( 'NONE', *, *, #6526, .F. ) ;
#9895=AXIS2_PLACEMENT_3D ( 'NONE', #7502, #1038, #9433 ) ;
#9911=ORIENTED_EDGE ( 'NONE', *, *, #44, .T. ) ;
#9916=DIRECTION ( 'NONE',  ( -0.000000000000000000, -1.000000000000000000, -0.000000000000000000 ) ) ;
#9922=VERTEX_POINT ( 'NONE', #8031 ) ;
#9930=CIRCLE ( 'NONE', #7087, 8.499999999999992895 ) ;
#9933=CARTESIAN_POINT ( 'NONE',  ( 0.8327827707325454742, 9.000000000000000000, 6.698430626405788679 ) ) ;
#9936=DIRECTION ( 'NONE',  ( -0.000000000000000000, 1.000000000000000000, -0.000000000000000000 ) ) ;
#9940=ORIENTED_EDGE ( 'NONE', *, *, #2697, .T. ) ;
#9946=CIRCLE ( 'NONE', #2479, 6.750000000000000888 ) ;
#9950=CARTESIAN_POINT ( 'NONE',  ( 6.749972395921142621, 9.000000000000000000, -0.01930425607464712062 ) ) ;
#9954=VECTOR ( 'NONE', #5575, 1000.000000000000000 ) ;
#9956=DIRECTION ( 'NONE',  ( 0.000000000000000000, 0.000000000000000000, -1.000000000000000000 ) ) ;
#9969=ORIENTED_EDGE ( 'NONE', *, *, #3182, .F. ) ;
#9974=CARTESIAN_POINT ( 'NONE',  ( -5.976238463952679325, 9.000000000000000000, -3.138004751744734477 ) ) ;
#9981=ORIENTED_EDGE ( 'NONE', *, *, #3952, .T. ) ;
#9988=AXIS2_PLACEMENT_3D ( 'NONE', #7862, #4839, #12083 ) ;
#9990=FILL_AREA_STYLE_COLOUR ( '', #9358 ) ;
#10000=ADVANCED_BREP_SHAPE_REPRESENTATION ( '', ( #13416, #10007 ), #6493 ) ;
#10002=AXIS2_PLACEMENT_3D ( 'NONE', #989, #9390, #8336 ) ;
#10003=ORIENTED_EDGE ( 'NONE', *, *, #1276, .F. ) ;
#10006=CARTESIAN_POINT ( 'NONE',  ( 7.248474140376192310, 9.000000000000000000, 4.439552076088041588 ) ) ;
#10007=AXIS2_PLACEMENT_3D ( 'NONE', #6754, #3381, #5712 ) ;
#10009=DIRECTION ( 'NONE',  ( 0.000000000000000000, 0.000000000000000000, 1.000000000000000000 ) ) ;
#10015=DIRECTION ( 'NONE',  ( 0.000000000000000000, 0.000000000000000000, 1.000000000000000000 ) ) ;
#10017=DIRECTION ( 'NONE',  ( 0.000000000000000000, 0.000000000000000000, -1.000000000000000000 ) ) ;
#10024=CARTESIAN_POINT ( 'NONE',  ( 0.000000000000000000, 9.000000000000000000, 0.000000000000000000 ) ) ;
#10025=EDGE_CURVE ( 'NONE', #10192, #11905, #5128, .T. ) ;
#10029=DIRECTION ( 'NONE',  ( 0.000000000000000000, 1.000000000000000000, -0.000000000000000000 ) ) ;
#10035=CYLINDRICAL_SURFACE ( 'NONE', #2269, 8.499999999999998224 ) ;
#10047=CARTESIAN_POINT ( 'NONE',  ( -5.830003112347290184, 9.000000000000000000, -5.394061460138155795 ) ) ;
#10052=ORIENTED_EDGE ( 'NONE', *, *, #11441, .F. ) ;
#10058=ORIENTED_EDGE ( 'NONE', *, *, #6082, .T. ) ;
#10060=VERTEX_POINT ( 'NONE', #11410 ) ;
#10061=DIRECTION ( 'NONE',  ( 0.000000000000000000, 0.000000000000000000, -1.000000000000000000 ) ) ;
#10064=CARTESIAN_POINT ( 'NONE',  ( -5.065227977808753224, 0.000000000000000000, -4.461610195077944319 ) ) ;
#10065=CARTESIAN_POINT ( 'NONE',  ( -0.7527353566742582824, 0.000000000000000000, 7.906594341344654886 ) ) ;
#10066=CARTESIAN_POINT ( 'NONE',  ( -3.533475733155565290, 9.000000000000000000, 7.730753471893975437 ) ) ;
#10067=ORIENTED_EDGE ( 'NONE', *, *, #2302, .T. ) ;
#10070=VECTOR ( 'NONE', #13231, 1000.000000000000000 ) ;
#10075=DIRECTION ( 'NONE',  ( 0.000000000000000000, 0.000000000000000000, 1.000000000000000000 ) ) ;
#10077=DIRECTION ( 'NONE',  ( 0.000000000000000000, 0.000000000000000000, 1.000000000000000000 ) ) ;
#10086=B_SPLINE_CURVE_WITH_KNOTS ( 'NONE', 3,
 ( #9028, #7122, #386, #4004 ),
 .UNSPECIFIED., .F., .F.,
 ( 4, 4 ),
 ( 0.000000000000000000, 0.8724294488011762327 ),
 .UNSPECIFIED. ) ;
#10088=ORIENTED_EDGE ( 'NONE', *, *, #3182, .T. ) ;
#10092=CARTESIAN_POINT ( 'NONE',  ( 0.000000000000000000, 9.000000000000000000, 0.000000000000000000 ) ) ;
#10100=DIRECTION ( 'NONE',  ( -0.000000000000000000, -1.000000000000000000, -0.000000000000000000 ) ) ;
#10102=AXIS2_PLACEMENT_3D ( 'NONE', #13210, #12266, #676 ) ;
#10105=LINE ( 'NONE', #1857, #9477 ) ;
#10106=CARTESIAN_POINT ( 'NONE',  ( -5.496871281090180972, 0.000000000000000000, 4.899765193453235135 ) ) ;
#10119=ORIENTED_EDGE ( 'NONE', *, *, #8274, .F. ) ;
#10128=CYLINDRICAL_SURFACE ( 'NONE', #11237, 6.750000000000000888 ) ;
#10133=CARTESIAN_POINT ( 'NONE',  ( 5.517918333394296049, 9.000000000000000000, 4.875228826198821253 ) ) ;
#10134=ORIENTED_EDGE ( 'NONE', *, *, #1555, .F. ) ;
#10136=CARTESIAN_POINT ( 'NONE',  ( 0.000000000000000000, 9.000000000000000000, 0.000000000000000000 ) ) ;
#10142=CARTESIAN_POINT ( 'NONE',  ( -0.8123631076467130452, 9.000000000000000000, -6.700937709107179785 ) ) ;
#10147=VECTOR ( 'NONE', #2439, 1000.000000000000000 ) ;
#10149=CARTESIAN_POINT ( 'NONE',  ( 3.007863545083557355, 0.000000000000000000, 7.350755164602351677 ) ) ;
#10151=LINE ( 'NONE', #12380, #5137 ) ;
#10157=AXIS2_PLACEMENT_3D ( 'NONE', #2139, #6544, #10744 ) ;
#10164=CIRCLE ( 'NONE', #4441, 9.250000000000000000 ) ;
#10172=FACE_OUTER_BOUND ( 'NONE', #220, .T. ) ;
#10184=FACE_OUTER_BOUND ( 'NONE', #9714, .T. ) ;
#10185=DIRECTION ( 'NONE',  ( 0.000000000000000000, 0.000000000000000000, 1.000000000000000000 ) ) ;
#10188=CARTESIAN_POINT ( 'NONE',  ( 6.736042615721505200, 0.000000000000000000, 5.184180733653466433 ) ) ;
#10190=AXIS2_PLACEMENT_3D ( 'NONE', #10324, #1865, #13501 ) ;
#10192=VERTEX_POINT ( 'NONE', #4034 ) ;
#10194=CARTESIAN_POINT ( 'NONE',  ( -6.721397655168932062, 9.000000000000000000, 5.203154193476253297 ) ) ;
#10210=CARTESIAN_POINT ( 'NONE',  ( 1.127406311874972422, 0.000000000000000000, -7.862174656777307646 ) ) ;
#10225=LINE ( 'NONE', #6024, #9459 ) ;
#10240=ORIENTED_EDGE ( 'NONE', *, *, #6320, .T. ) ;
#10245=CARTESIAN_POINT ( 'NONE',  ( 5.967832595844252630, 9.000000000000000000, -3.153961652902406154 ) ) ;
#10249=CARTESIAN_POINT ( 'NONE',  ( 0.000000000000000000, 0.000000000000000000, 0.000000000000000000 ) ) ;
#10251=CARTESIAN_POINT ( 'NONE',  ( -5.977417671213808070, 9.000000000000000000, 3.135757960025116642 ) ) ;
#10252=CARTESIAN_POINT ( 'NONE',  ( 4.369710415961185035, 9.000000000000000000, 6.632530905044255576 ) ) ;
#10267=CARTESIAN_POINT ( 'NONE',  ( 0.000000000000000000, 0.000000000000000000, 0.000000000000000000 ) ) ;
#10276=ORIENTED_EDGE ( 'NONE', *, *, #4134, .F. ) ;
#10280=EDGE_CURVE ( 'NONE', #912, #5239, #9316, .T. ) ;
#10294=ORIENTED_EDGE ( 'NONE', *, *, #290, .F. ) ;
#10298=VERTEX_POINT ( 'NONE', #8557 ) ;
#10300=ADVANCED_FACE ( 'NONE', ( #10651 ), #7858, .T. ) ;
#10301=ADVANCED_FACE ( 'NONE', ( #7807 ), #3454, .T. ) ;
#10302=ORIENTED_EDGE ( 'NONE', *, *, #10025, .T. ) ;
#10309=ADVANCED_FACE ( 'NONE', ( #12028 ), #11823, .T. ) ;
#10313=CARTESIAN_POINT ( 'NONE',  ( -6.749999880766614169, 9.000000000000000000, -0.001268720102703135150 ) ) ;
#10316=DIRECTION ( 'NONE',  ( 0.000000000000000000, 0.000000000000000000, 1.000000000000000000 ) ) ;
#10324=CARTESIAN_POINT ( 'NONE',  ( 0.000000000000000000, 9.000000000000000000, 0.000000000000000000 ) ) ;
#10328=AXIS2_PLACEMENT_3D ( 'NONE', #1368, #4673, #404 ) ;
#10329=VERTEX_POINT ( 'NONE', #8970 ) ;
#10330=CARTESIAN_POINT ( 'NONE',  ( 6.736042615721505200, 9.000000000000000000, 5.184180733653466433 ) ) ;
#10332=FACE_OUTER_BOUND ( 'NONE', #9799, .T. ) ;
#10333=LINE ( 'NONE', #11376, #1635 ) ;
#10343=ORIENTED_EDGE ( 'NONE', *, *, #11635, .T. ) ;
#10347=CARTESIAN_POINT ( 'NONE',  ( -6.057461899949976747, 0.000000000000000000, 5.137313564148215939 ) ) ;
#10350=EDGE_CURVE ( 'NONE', #7728, #1004, #6303, .T. ) ;
#10363=ORIENTED_EDGE ( 'NONE', *, *, #12727, .F. ) ;
#10368=CIRCLE ( 'NONE', #2225, 8.500000000000001776 ) ;
#10371=CARTESIAN_POINT ( 'NONE',  ( 7.146769547044127258, -1.694065894508600678E-18, -1.771712133291270863 ) ) ;
#10372=DIRECTION ( 'NONE',  ( -0.000000000000000000, 1.000000000000000000, -0.000000000000000000 ) ) ;
#10379=ORIENTED_EDGE ( 'NONE', *, *, #301, .F. ) ;
#10381=ORIENTED_EDGE ( 'NONE', *, *, #11088, .F. ) ;
#10394=ORIENTED_EDGE ( 'NONE', *, *, #3165, .T. ) ;
#10414=VERTEX_POINT ( 'NONE', #650 ) ;
#10417=VERTEX_POINT ( 'NONE', #3669 ) ;
#10431=CARTESIAN_POINT ( 'NONE',  ( 0.000000000000000000, 0.000000000000000000, 0.000000000000000000 ) ) ;
#10456=DIRECTION ( 'NONE',  ( -0.000000000000000000, -1.000000000000000000, -0.000000000000000000 ) ) ;
#10457=ORIENTED_EDGE ( 'NONE', *, *, #7248, .T. ) ;
#10465=CARTESIAN_POINT ( 'NONE',  ( -6.749999880766614169, 1.734723475976807094E-15, -0.001268720102703522860 ) ) ;
#10475=ORIENTED_EDGE ( 'NONE', *, *, #6318, .T. ) ;
#10485=DIRECTION ( 'NONE',  ( 0.000000000000000000, 1.000000000000000000, -0.000000000000000000 ) ) ;
#10490=CARTESIAN_POINT ( 'NONE',  ( 2.394769219159762041, 9.000000000000000000, -6.310909632292713844 ) ) ;
#10502=CARTESIAN_POINT ( 'NONE',  ( -5.976238463952679325, 9.000000000000000000, -3.138004751744734477 ) ) ;
#10503=B_SPLINE_SURFACE_WITH_KNOTS ( 'NONE', 3, 1, ( 
 ( #32, #9322 ),
 ( #12509, #5193 ),
 ( #2917, #4209 ),
 ( #9392, #920 ) ),
 .UNSPECIFIED., .F., .F., .F.,
 ( 4, 4 ),
 ( 2, 2 ),
 ( 0.1276832474596253097, 1.000000000000000000 ),
 ( 0.000000000000000000, 1.000000000000000000 ),
 .UNSPECIFIED. ) ;
#10515=DIRECTION ( 'NONE',  ( 0.000000000000000000, 0.000000000000000000, -1.000000000000000000 ) ) ;
#10516=VERTEX_POINT ( 'NONE', #7132 ) ;
#10525=DIRECTION ( 'NONE',  ( -0.000000000000000000, -1.000000000000000000, -0.000000000000000000 ) ) ;
#10527=EDGE_CURVE ( 'NONE', #8800, #9922, #9880, .T. ) ;
#10528=LINE ( 'NONE', #11765, #8878 ) ;
#10544=CARTESIAN_POINT ( 'NONE',  ( -3.533475733155563070, 0.000000000000000000, 7.730753471893976325 ) ) ;
#10554=CARTESIAN_POINT ( 'NONE',  ( 7.659717769608228366, 9.000000000000000000, -2.099897208369672530 ) ) ;
#10555=ORIENTED_EDGE ( 'NONE', *, *, #3411, .F. ) ;
#10556=B_SPLINE_CURVE_WITH_KNOTS ( 'NONE', 3,
 ( #4897, #9097, #778, #7792 ),
 .UNSPECIFIED., .F., .F.,
 ( 4, 4 ),
 ( 0.000000000000000000, 0.8724294488011763438 ),
 .UNSPECIFIED. ) ;
#10569=APPLICATION_CONTEXT ( 'automotive_design' ) ;
#10572=CARTESIAN_POINT ( 'NONE',  ( 4.201465772524378472, 0.000000000000000000, 6.047394330962382547 ) ) ;
#10584=VERTEX_POINT ( 'NONE', #4150 ) ;
#10585=CARTESIAN_POINT ( 'NONE',  ( 4.369710415961185035, 9.000000000000000000, 6.632530905044255576 ) ) ;
#10591=PLANE ( 'NONE',  #11678 ) ;
#10606=CARTESIAN_POINT ( 'NONE',  ( -7.235926821844434365, 0.000000000000000000, 4.459973433655444630 ) ) ;
#10609=FACE_OUTER_BOUND ( 'NONE', #2324, .T. ) ;
#10615=CIRCLE ( 'NONE', #11053, 8.500000000000000000 ) ;
#10621=ORIENTED_EDGE ( 'NONE', *, *, #9798, .F. ) ;
#10623=ADVANCED_FACE ( 'NONE', ( #13595 ), #6649, .T. ) ;
#10637=LINE ( 'NONE', #5122, #4292 ) ;
#10639=CARTESIAN_POINT ( 'NONE',  ( 5.053288777954491273, 0.000000000000000000, -4.475128213425755952 ) ) ;
#10641=ORIENTED_EDGE ( 'NONE', *, *, #737, .F. ) ;
#10645=B_SPLINE_CURVE_WITH_KNOTS ( 'NONE', 3,
 ( #1625, #13339, #2786, #7875 ),
 .UNSPECIFIED., .F., .F.,
 ( 4, 4 ),
 ( 0.1276832474596284739, 1.000000000000000000 ),
 .UNSPECIFIED. ) ;
#10647=CARTESIAN_POINT ( 'NONE',  ( -5.977417671213808070, 9.000000000000000000, 3.135757960025116642 ) ) ;
#10649=EDGE_CURVE ( 'NONE', #7402, #5243, #1194, .T. ) ;
#10650=CIRCLE ( 'NONE', #12134, 6.749999999999999112 ) ;
#10651=FACE_OUTER_BOUND ( 'NONE', #3073, .T. ) ;
#10655=DIRECTION ( 'NONE',  ( -0.000000000000000000, -1.000000000000000000, -0.000000000000000000 ) ) ;
#10672=DIRECTION ( 'NONE',  ( 0.000000000000000000, 0.000000000000000000, -1.000000000000000000 ) ) ;
#10684=CARTESIAN_POINT ( 'NONE',  ( -5.299649803506881085, 9.000000000000000000, -6.645578376649351249 ) ) ;
#10703=ADVANCED_FACE ( 'NONE', ( #9595 ), #368, .T. ) ;
#10712=CARTESIAN_POINT ( 'NONE',  ( -8.369528376005813897, 0.000000000000000000, 1.483574994138652903 ) ) ;
#10721=CARTESIAN_POINT ( 'NONE',  ( -5.977417671213808070, 9.000000000000000000, 3.135757960025116642 ) ) ;
#10725=CARTESIAN_POINT ( 'NONE',  ( 0.000000000000000000, 9.000000000000000000, 0.000000000000000000 ) ) ;
#10735=ORIENTED_EDGE ( 'NONE', *, *, #490, .T. ) ;
#10744=DIRECTION ( 'NONE',  ( 0.000000000000000000, 0.000000000000000000, 1.000000000000000000 ) ) ;
#10748=ORIENTED_EDGE ( 'NONE', *, *, #7345, .F. ) ;
#10750=AXIS2_PLACEMENT_3D ( 'NONE', #1937, #11307, #9298 ) ;
#10753=ORIENTED_EDGE ( 'NONE', *, *, #4748, .T. ) ;
#10756=CARTESIAN_POINT ( 'NONE',  ( -4.334442004268530546, 0.000000000000000000, 7.311813216407585081 ) ) ;
#10759=CARTESIAN_POINT ( 'NONE',  ( -0.7527353566742582824, 9.000000000000000000, 7.906594341344654886 ) ) ;
#10761=VERTEX_POINT ( 'NONE', #10064 ) ;
#10768=CARTESIAN_POINT ( 'NONE',  ( 6.553553527263006551, 9.000000000000000000, 1.616612558808879774 ) ) ;
#10771=CARTESIAN_POINT ( 'NONE',  ( 7.940744365623959133, 0.000000000000000000, 0.1715058177969961128 ) ) ;
#10777=ORIENTED_EDGE ( 'NONE', *, *, #10916, .F. ) ;
#10782=CARTESIAN_POINT ( 'NONE',  ( 5.967832595844251742, 9.000000000000000000, -3.153961652902404822 ) ) ;
#10785=EDGE_CURVE ( 'NONE', #8580, #11681, #8439, .T. ) ;
#10786=FACE_OUTER_BOUND ( 'NONE', #11020, .T. ) ;
#10801=EDGE_CURVE ( 'NONE', #2415, #4379, #10556, .T. ) ;
#10803=DIRECTION ( 'NONE',  ( -0.000000000000000000, -1.000000000000000000, -0.000000000000000000 ) ) ;
#10805=CARTESIAN_POINT ( 'NONE',  ( 5.053288777954493050, 9.000000000000000000, -4.475128213425755952 ) ) ;
#10809=VERTEX_POINT ( 'NONE', #12009 ) ;
#10816=ADVANCED_FACE ( 'NONE', ( #12141 ), #4769, .T. ) ;
#10818=ORIENTED_EDGE ( 'NONE', *, *, #2310, .T. ) ;
#10828=AXIS2_PLACEMENT_3D ( 'NONE', #7546, #8631, #12980 ) ;
#10830=CARTESIAN_POINT ( 'NONE',  ( -4.340891659662447388, 9.000000000000000000, 6.651128039276029469 ) ) ;
#10845=CARTESIAN_POINT ( 'NONE',  ( -8.479748006907129820, 0.000000000000000000, 0.5864074857593144507 ) ) ;
#10853=EDGE_LOOP ( 'NONE', ( #12278, #9514, #5762, #12242 ) ) ;
#10857=PRODUCT ( 'base-gear', 'base-gear', '', ( #8310 ) ) ;
#10862=CARTESIAN_POINT ( 'NONE',  ( 0.8653219153705552502, 0.000000000000000000, -7.312626806738413698 ) ) ;
#10868=AXIS2_PLACEMENT_3D ( 'NONE', #451, #2588, #8839 ) ;
#10869=CIRCLE ( 'NONE', #8651, 6.749999999999999112 ) ;
#10875=EDGE_CURVE ( 'NONE', #8580, #12645, #10333, .T. ) ;
#10894=CARTESIAN_POINT ( 'NONE',  ( 0.7944557581062196006, 9.000000000000000000, -6.703084368289862205 ) ) ;
#10898=CARTESIAN_POINT ( 'NONE',  ( 1.580708947611199511, 9.000000000000000000, -8.351727918397596540 ) ) ;
#10905=ORIENTED_EDGE ( 'NONE', *, *, #12810, .T. ) ;
#10916=EDGE_CURVE ( 'NONE', #1554, #76, #10869, .T. ) ;
#10935=ORIENTED_EDGE ( 'NONE', *, *, #1698, .T. ) ;
#10940=PRODUCT_DEFINITION ( 'UNKNOWN', '', #2999, #6686 ) ;
#10947=CARTESIAN_POINT ( 'NONE',  ( 3.555260608155774271, 9.000000000000000000, 7.720759160088842776 ) ) ;
#10955=ORIENTED_EDGE ( 'NONE', *, *, #1796, .F. ) ;
#10959=LINE ( 'NONE', #5866, #3522 ) ;
#10965=EDGE_LOOP ( 'NONE', ( #7509, #10294, #4095, #4946 ) ) ;
#10971=EDGE_CURVE ( 'NONE', #11905, #11924, #2197, .T. ) ;
#10979=CARTESIAN_POINT ( 'NONE',  ( 3.555260608155774271, 9.000000000000000000, 7.720759160088842776 ) ) ;
#10980=CYLINDRICAL_SURFACE ( 'NONE', #80, 6.750000000000000888 ) ;
#10983=AXIS2_PLACEMENT_3D ( 'NONE', #9148, #615, #10316 ) ;
#10988=DIRECTION ( 'NONE',  ( 0.000000000000000000, 0.000000000000000000, -1.000000000000000000 ) ) ;
#10990=CARTESIAN_POINT ( 'NONE',  ( 5.280889752749253319, 0.000000000000000000, -6.660495733750448899 ) ) ;
#10996=EDGE_LOOP ( 'NONE', ( #13324, #1763, #5519, #5904 ) ) ;
#10997=ORIENTED_EDGE ( 'NONE', *, *, #13353, .F. ) ;
#11007=CYLINDRICAL_SURFACE ( 'NONE', #6178, 6.750000000000000888 ) ;
#11016=VERTEX_POINT ( 'NONE', #12745 ) ;
#11019=DIRECTION ( 'NONE',  ( 0.000000000000000000, 0.000000000000000000, 1.000000000000000000 ) ) ;
#11020=EDGE_LOOP ( 'NONE', ( #789, #4974, #3868, #6280 ) ) ;
#11023=DIRECTION ( 'NONE',  ( 0.000000000000000000, 0.000000000000000000, 1.000000000000000000 ) ) ;
#11027=CARTESIAN_POINT ( 'NONE',  ( -5.975392301194336397, 9.000000000000000000, -6.045220165289885372 ) ) ;
#11030=CARTESIAN_POINT ( 'NONE',  ( -6.721397655168932062, 9.000000000000000000, 5.203154193476253297 ) ) ;
#11032=ADVANCED_FACE ( 'NONE', ( #9637 ), #154, .F. ) ;
#11033=VERTEX_POINT ( 'NONE', #1241 ) ;
#11034=EDGE_CURVE ( 'NONE', #4686, #2755, #5802, .T. ) ;
#11040=VECTOR ( 'NONE', #13485, 1000.000000000000000 ) ;
#11043=CARTESIAN_POINT ( 'NONE',  ( -3.833392836528145331, 1.734723475976807094E-15, -5.555861711818853799 ) ) ;
#11051=EDGE_CURVE ( 'NONE', #3124, #9464, #4541, .T. ) ;
#11053=AXIS2_PLACEMENT_3D ( 'NONE', #13372, #832, #11019 ) ;
#11061=AXIS2_PLACEMENT_3D ( 'NONE', #12327, #10100, #7890 ) ;
#11065=CARTESIAN_POINT ( 'NONE',  ( 5.280889752749253319, 9.000000000000000000, -6.660495733750448899 ) ) ;
#11073=ORIENTED_EDGE ( 'NONE', *, *, #7340, .F. ) ;
#11077=AXIS2_PLACEMENT_3D ( 'NONE', #3485, #3625, #6661 ) ;
#11081=DIRECTION ( 'NONE',  ( 0.000000000000000000, 0.000000000000000000, 1.000000000000000000 ) ) ;
#11088=EDGE_CURVE ( 'NONE', #7728, #4686, #214, .T. ) ;
#11090=CARTESIAN_POINT ( 'NONE',  ( 0.000000000000000000, 9.000000000000000000, 0.000000000000000000 ) ) ;
#11093=DIRECTION ( 'NONE',  ( 0.000000000000000000, 1.000000000000000000, -0.000000000000000000 ) ) ;
#11097=AXIS2_PLACEMENT_3D ( 'NONE', #960, #12539, #1990 ) ;
#11107=ORIENTED_EDGE ( 'NONE', *, *, #4654, .T. ) ;
#11108=( GEOMETRIC_REPRESENTATION_CONTEXT ( 3 ) GLOBAL_UNCERTAINTY_ASSIGNED_CONTEXT ( ( #8185 ) ) GLOBAL_UNIT_ASSIGNED_CONTEXT ( ( #1954, #6019, #8080 ) ) REPRESENTATION_CONTEXT ( 'NONE', 'WORKASPACE' ) );
#11116=AXIS2_PLACEMENT_3D ( 'NONE', #4878, #1660, #476 ) ;
#11121=CARTESIAN_POINT ( 'NONE',  ( -4.190859029938718727, 9.000000000000000000, -6.054087828318142073 ) ) ;
#11123=EDGE_CURVE ( 'NONE', #7795, #8354, #11309, .T. ) ;
#11129=EDGE_LOOP ( 'NONE', ( #9862, #9889, #10955, #1181 ) ) ;
#11139=FACE_OUTER_BOUND ( 'NONE', #12503, .T. ) ;
#11140=EDGE_CURVE ( 'NONE', #7190, #3870, #6947, .T. ) ;
#11148=EDGE_CURVE ( 'NONE', #11016, #5839, #1349, .T. ) ;
#11152=CYLINDRICAL_SURFACE ( 'NONE', #2213, 8.500000000000000000 ) ;
#11178=VERTEX_POINT ( 'NONE', #12055 ) ;
#11181=CARTESIAN_POINT ( 'NONE',  ( 5.985774866078160450, 0.000000000000000000, 3.119775513178307147 ) ) ;
#11186=CARTESIAN_POINT ( 'NONE',  ( 0.9098489087730803337, 9.000000000000000000, 7.307220250892556557 ) ) ;
#11190=DIRECTION ( 'NONE',  ( -0.000000000000000000, -1.000000000000000000, -0.000000000000000000 ) ) ;
#11192=VERTEX_POINT ( 'NONE', #1448 ) ;
#11211=EDGE_CURVE ( 'NONE', #912, #3761, #13348, .T. ) ;
#11212=AXIS2_PLACEMENT_3D ( 'NONE', #13493, #7161, #11360 ) ;
#11217=LINE ( 'NONE', #13565, #5160 ) ;
#11219=CARTESIAN_POINT ( 'NONE',  ( -0.8123631076467130452, 9.000000000000000000, -6.700937709107178009 ) ) ;
#11220=VERTEX_POINT ( 'NONE', #5848 ) ;
#11225=AXIS2_PLACEMENT_3D ( 'NONE', #647, #3732, #4447 ) ;
#11237=AXIS2_PLACEMENT_3D ( 'NONE', #5099, #9165, #6072 ) ;
#11239=CARTESIAN_POINT ( 'NONE',  ( 0.7944557581062193785, 0.000000000000000000, -6.703084368289860429 ) ) ;
#11242=CARTESIAN_POINT ( 'NONE',  ( 0.000000000000000000, 0.000000000000000000, 0.000000000000000000 ) ) ;
#11246=ORIENTED_EDGE ( 'NONE', *, *, #12727, .T. ) ;
#11247=FACE_OUTER_BOUND ( 'NONE', #4316, .T. ) ;
#11255=CARTESIAN_POINT ( 'NONE',  ( -0.4399887592034530392, 0.000000000000000000, 8.488604708182295511 ) ) ;
#11265=CIRCLE ( 'NONE', #8398, 6.750000000000000888 ) ;
#11271=DIRECTION ( 'NONE',  ( 0.000000000000000000, 0.000000000000000000, 1.000000000000000000 ) ) ;
#11276=AXIS2_PLACEMENT_3D ( 'NONE', #4956, #10655, #3610 ) ;
#11284=AXIS2_PLACEMENT_3D ( 'NONE', #5829, #10029, #600 ) ;
#11286=DIRECTION ( 'NONE',  ( -0.000000000000000000, -1.000000000000000000, -0.000000000000000000 ) ) ;
#11289=CARTESIAN_POINT ( 'NONE',  ( 0.000000000000000000, 9.000000000000000000, 0.000000000000000000 ) ) ;
#11301=CIRCLE ( 'NONE', #296, 6.750000000000000888 ) ;
#11307=DIRECTION ( 'NONE',  ( 0.000000000000000000, 1.000000000000000000, -0.000000000000000000 ) ) ;
#11309=CIRCLE ( 'NONE', #5358, 6.750000000000000888 ) ;
#11325=CARTESIAN_POINT ( 'NONE',  ( -1.604252589105048976, 9.000000000000000000, -8.347237484961699039 ) ) ;
#11327=CARTESIAN_POINT ( 'NONE',  ( 4.652003457867571967, 9.000000000000000000, -6.437678087145717321 ) ) ;
#11333=AXIS2_PLACEMENT_3D ( 'NONE', #10431, #2159, #5320 ) ;
#11339=VERTEX_POINT ( 'NONE', #4181 ) ;
#11345=EDGE_CURVE ( 'NONE', #12325, #7402, #3837, .T. ) ;
#11349=CARTESIAN_POINT ( 'NONE',  ( -0.8148820470561124463, 0.000000000000000000, 6.700631854488474204 ) ) ;
#11357=B_SPLINE_CURVE_WITH_KNOTS ( 'NONE', 3,
 ( #5593, #10830, #6627, #3390 ),
 .UNSPECIFIED., .F., .F.,
 ( 4, 4 ),
 ( 0.1276832474596244493, 1.000000000000000000 ),
 .UNSPECIFIED. ) ;
#11360=DIRECTION ( 'NONE',  ( 0.000000000000000000, 0.000000000000000000, -1.000000000000000000 ) ) ;
#11366=B_SPLINE_SURFACE_WITH_KNOTS ( 'NONE', 3, 1, ( 
 ( #2321, #1341 ),
 ( #12722, #5469 ),
 ( #10585, #3471 ),
 ( #8501, #9676 ) ),
 .UNSPECIFIED., .F., .F., .F.,
 ( 4, 4 ),
 ( 2, 2 ),
 ( 0.000000000000000000, 0.8724294488011777871 ),
 ( 0.000000000000000000, 1.000000000000000000 ),
 .UNSPECIFIED. ) ;
#11374=CARTESIAN_POINT ( 'NONE',  ( 2.392396671352951198, 9.000000000000000000, 6.311809420990095454 ) ) ;
#11376=CARTESIAN_POINT ( 'NONE',  ( 8.093005444143644311, 9.000000000000000000, -2.598704077239528232 ) ) ;
#11379=ORIENTED_EDGE ( 'NONE', *, *, #7702, .F. ) ;
#11384=EDGE_CURVE ( 'NONE', #10060, #3498, #11217, .T. ) ;
#11397=CARTESIAN_POINT ( 'NONE',  ( 2.392396671352951198, 0.000000000000000000, 6.311809420990095454 ) ) ;
#11410=CARTESIAN_POINT ( 'NONE',  ( -3.833392836528144443, 9.000000000000000000, -5.555861711818853799 ) ) ;
#11412=DIRECTION ( 'NONE',  ( 0.000000000000000000, 0.000000000000000000, 1.000000000000000000 ) ) ;
#11439=CIRCLE ( 'NONE', #6161, 6.750000000000000888 ) ;
#11441=EDGE_CURVE ( 'NONE', #7238, #9762, #4252, .T. ) ;
#11457=CARTESIAN_POINT ( 'NONE',  ( -4.334442004268525217, 9.000000000000000000, 7.311813216407587745 ) ) ;
#11460=ORIENTED_EDGE ( 'NONE', *, *, #2322, .F. ) ;
#11461=CARTESIAN_POINT ( 'NONE',  ( 0.000000000000000000, 9.000000000000000000, 0.000000000000000000 ) ) ;
#11469=CARTESIAN_POINT ( 'NONE',  ( -8.100301009650799244, 0.000000000000000000, -2.575873357339268033 ) ) ;
#11492=EDGE_CURVE ( 'NONE', #10414, #11737, #4386, .T. ) ;
#11493=DIRECTION ( 'NONE',  ( -0.000000000000000000, -1.000000000000000000, -0.000000000000000000 ) ) ;
#11499=ORIENTED_EDGE ( 'NONE', *, *, #5965, .T. ) ;
#11509=CIRCLE ( 'NONE', #952, 8.499999999999996447 ) ;
#11529=CARTESIAN_POINT ( 'NONE',  ( -7.125870497355421662, 0.000000000000000000, -3.507536778237742237 ) ) ;
#11531=B_SPLINE_CURVE_WITH_KNOTS ( 'NONE', 3,
 ( #10894, #13101, #5786, #2560 ),
 .UNSPECIFIED., .F., .F.,
 ( 4, 4 ),
 ( 0.000000000000000000, 0.8724294488011757887 ),
 .UNSPECIFIED. ) ;
#11535=CARTESIAN_POINT ( 'NONE',  ( -6.549210654805285081, 9.000000000000000000, 1.634117437329677180 ) ) ;
#11545=EDGE_CURVE ( 'NONE', #933, #11943, #10528, .T. ) ;
#11551=DIRECTION ( 'NONE',  ( 0.000000000000000000, 0.000000000000000000, -1.000000000000000000 ) ) ;
#11554=ORIENTED_EDGE ( 'NONE', *, *, #346, .T. ) ;
#11559=CARTESIAN_POINT ( 'NONE',  ( 4.355042381134426321, 9.000000000000000000, 7.299562031966228659 ) ) ;
#11562=ORIENTED_EDGE ( 'NONE', *, *, #1343, .T. ) ;
#11563=CARTESIAN_POINT ( 'NONE',  ( 3.850308450823737516, 9.000000000000000000, 5.544152309732777617 ) ) ;
#11581=CARTESIAN_POINT ( 'NONE',  ( -5.977417671213807182, 9.000000000000000000, 3.135757960025121527 ) ) ;
#11585=DIRECTION ( 'NONE',  ( -0.000000000000000000, -1.000000000000000000, -0.000000000000000000 ) ) ;
#11591=ORIENTED_EDGE ( 'NONE', *, *, #7611, .T. ) ;
#11619=ORIENTED_EDGE ( 'NONE', *, *, #2207, .T. ) ;
#11623=FACE_OUTER_BOUND ( 'NONE', #13074, .T. ) ;
#11627=CIRCLE ( 'NONE', #10750, 6.750000000000000888 ) ;
#11629=ADVANCED_FACE ( 'NONE', ( #11139 ), #4674, .T. ) ;
#11635=EDGE_CURVE ( 'NONE', #12802, #7012, #3684, .T. ) ;
#11652=CARTESIAN_POINT ( 'NONE',  ( 7.146769547044127258, 9.000000000000000000, -1.771712133291270863 ) ) ;
#11663=EDGE_CURVE ( 'NONE', #8976, #11033, #3309, .T. ) ;
#11668=ORIENTED_EDGE ( 'NONE', *, *, #125, .F. ) ;
#11678=AXIS2_PLACEMENT_3D ( 'NONE', #6723, #4450, #6584 ) ;
#11681=VERTEX_POINT ( 'NONE', #9057 ) ;
#11709=EDGE_CURVE ( 'NONE', #672, #4801, #12571, .T. ) ;
#11713=CIRCLE ( 'NONE', #6870, 8.500000000000000000 ) ;
#11723=B_SPLINE_CURVE_WITH_KNOTS ( 'NONE', 3,
 ( #8305, #1851, #10252, #11559 ),
 .UNSPECIFIED., .F., .F.,
 ( 4, 4 ),
 ( 0.000000000000000000, 0.8724294488011777871 ),
 .UNSPECIFIED. ) ;
#11730=CARTESIAN_POINT ( 'NONE',  ( 7.771282357155271825, 0.000000000000000000, -3.443424244174282389 ) ) ;
#11734=EDGE_CURVE ( 'NONE', #8800, #8278, #2746, .T. ) ;
#11737=VERTEX_POINT ( 'NONE', #6425 ) ;
#11746=CARTESIAN_POINT ( 'NONE',  ( 2.601737331980797041, -1.694065894508600678E-18, -6.888123234756056590 ) ) ;
#11748=CARTESIAN_POINT ( 'NONE',  ( -6.749999880766614169, 0.000000000000000000, -0.001268720102703522860 ) ) ;
#11755=DIRECTION ( 'NONE',  ( -0.000000000000000000, -1.000000000000000000, -0.000000000000000000 ) ) ;
#11760=DIRECTION ( 'NONE',  ( 0.000000000000000000, 0.000000000000000000, 1.000000000000000000 ) ) ;
#11761=CARTESIAN_POINT ( 'NONE',  ( 6.509732753943064054, 9.000000000000000000, -3.441899519755141412 ) ) ;
#11764=STYLED_ITEM('',(#13628),#13416);
#11765=CARTESIAN_POINT ( 'NONE',  ( 0.7944557581062196006, 9.000000000000000000, -6.703084368289862205 ) ) ;
#11778=DIRECTION ( 'NONE',  ( 0.000000000000000000, 0.000000000000000000, 1.000000000000000000 ) ) ;
#11786=EDGE_LOOP ( 'NONE', ( #7931, #4137, #12578, #2595 ) ) ;
#11787=ORIENTED_EDGE ( 'NONE', *, *, #24, .T. ) ;
#11792=VERTEX_POINT ( 'NONE', #4153 ) ;
#11795=ORIENTED_EDGE ( 'NONE', *, *, #7, .T. ) ;
#11796=PRESENTATION_STYLE_ASSIGNMENT (( #9848 ) ) ;
#11804=EDGE_CURVE ( 'NONE', #4379, #2013, #10637, .T. ) ;
#11809=ORIENTED_EDGE ( 'NONE', *, *, #11663, .F. ) ;
#11812=B_SPLINE_CURVE_WITH_KNOTS ( 'NONE', 3,
 ( #1177, #12888, #12621, #10544 ),
 .UNSPECIFIED., .F., .F.,
 ( 4, 4 ),
 ( 0.000000000000000000, 0.8724294488011768989 ),
 .UNSPECIFIED. ) ;
#11823=B_SPLINE_SURFACE_WITH_KNOTS ( 'NONE', 3, 1, ( 
 ( #9608, #12779 ),
 ( #184, #380 ),
 ( #6571, #5670 ),
 ( #4436, #10712 ) ),
 .UNSPECIFIED., .F., .F., .F.,
 ( 4, 4 ),
 ( 2, 2 ),
 ( 0.000000000000000000, 0.8724294488011786752 ),
 ( 0.000000000000000000, 1.000000000000000000 ),
 .UNSPECIFIED. ) ;
#11827=CYLINDRICAL_SURFACE ( 'NONE', #11225, 8.499999999999996447 ) ;
#11832=EDGE_CURVE ( 'NONE', #3124, #11905, #11357, .T. ) ;
#11837=ORIENTED_EDGE ( 'NONE', *, *, #11123, .T. ) ;
#11842=ORIENTED_EDGE ( 'NONE', *, *, #4467, .T. ) ;
#11844=CARTESIAN_POINT ( 'NONE',  ( 7.659717769608228366, 9.000000000000000000, -2.099897208369672530 ) ) ;
#11847=CARTESIAN_POINT ( 'NONE',  ( -6.721397655168932062, 9.000000000000000000, 5.203154193476253297 ) ) ;
#11856=ORIENTED_EDGE ( 'NONE', *, *, #5677, .T. ) ;
#11863=CARTESIAN_POINT ( 'NONE',  ( -0.8776997859584816375, 9.000000000000000000, 7.310603390113379341 ) ) ;
#11866=CARTESIAN_POINT ( 'NONE',  ( 5.806472362263156661, 0.000000000000000000, -5.419014975255640465 ) ) ;
#11867=ORIENTED_EDGE ( 'NONE', *, *, #8509, .T. ) ;
#11871=DIRECTION ( 'NONE',  ( -0.000000000000000000, -1.000000000000000000, -0.000000000000000000 ) ) ;
#11877=CARTESIAN_POINT ( 'NONE',  ( 2.392396671352952087, 9.000000000000000000, 6.311809420990097230 ) ) ;
#11890=B_SPLINE_SURFACE_WITH_KNOTS ( 'NONE', 3, 1, ( 
 ( #5527, #9604 ),
 ( #2372, #6567 ),
 ( #182, #7667 ),
 ( #10768, #2432 ) ),
 .UNSPECIFIED., .F., .F., .F.,
 ( 4, 4 ),
 ( 2, 2 ),
 ( 0.1276832474596280298, 1.000000000000000000 ),
 ( 0.000000000000000000, 1.000000000000000000 ),
 .UNSPECIFIED. ) ;
#11892=DIRECTION ( 'NONE',  ( 0.000000000000000000, 1.000000000000000000, -0.000000000000000000 ) ) ;
#11898=B_SPLINE_CURVE_WITH_KNOTS ( 'NONE', 3,
 ( #9300, #7179, #9226, #6267 ),
 .UNSPECIFIED., .F., .F.,
 ( 4, 4 ),
 ( 0.1276832474596280298, 1.000000000000000000 ),
 .UNSPECIFIED. ) ;
#11899=CARTESIAN_POINT ( 'NONE',  ( -5.039625798601655937, 0.000000000000000000, 4.490509081392509927 ) ) ;
#11905=VERTEX_POINT ( 'NONE', #4360 ) ;
#11911=VECTOR ( 'NONE', #1686, 1000.000000000000000 ) ;
#11914=DIRECTION ( 'NONE',  ( -0.000000000000000000, -1.000000000000000000, -0.000000000000000000 ) ) ;
#11923=AXIS2_PLACEMENT_3D ( 'NONE', #3927, #4972, #4197 ) ;
#11924=VERTEX_POINT ( 'NONE', #9722 ) ;
#11926=VERTEX_POINT ( 'NONE', #13033 ) ;
#11928=FACE_OUTER_BOUND ( 'NONE', #4046, .T. ) ;
#11931=FACE_OUTER_BOUND ( 'NONE', #2888, .T. ) ;
#11943=VERTEX_POINT ( 'NONE', #13381 ) ;
#11947=CARTESIAN_POINT ( 'NONE',  ( -2.411622991978541464, 0.000000000000000000, -6.304488444319688689 ) ) ;
#11951=DIRECTION ( 'NONE',  ( 0.000000000000000000, 0.000000000000000000, 1.000000000000000000 ) ) ;
#11979=ORIENTED_EDGE ( 'NONE', *, *, #10971, .T. ) ;
#11998=STYLED_ITEM ( 'NONE', ( #11796 ), #10000 ) ;
#11999=ORIENTED_EDGE ( 'NONE', *, *, #792, .T. ) ;
#12001=CYLINDRICAL_SURFACE ( 'NONE', #7536, 6.750000000000000888 ) ;
#12009=CARTESIAN_POINT ( 'NONE',  ( -5.975392301194336397, 0.000000000000000000, -6.045220165289885372 ) ) ;
#12016=ORIENTED_EDGE ( 'NONE', *, *, #5793, .T. ) ;
#12022=LINE ( 'NONE', #10502, #8834 ) ;
#12028=FACE_OUTER_BOUND ( 'NONE', #12148, .T. ) ;
#12033=ORIENTED_EDGE ( 'NONE', *, *, #2302, .F. ) ;
#12038=CARTESIAN_POINT ( 'NONE',  ( 0.7944557581062194895, 0.000000000000000000, -6.703084368289861317 ) ) ;
#12043=CARTESIAN_POINT ( 'NONE',  ( 0.000000000000000000, 9.000000000000000000, 0.000000000000000000 ) ) ;
#12047=VERTEX_POINT ( 'NONE', #10066 ) ;
#12052=FACE_OUTER_BOUND ( 'NONE', #5939, .T. ) ;
#12055=CARTESIAN_POINT ( 'NONE',  ( 2.392396671352952087, 9.000000000000000000, 6.311809420990097230 ) ) ;
#12064=ORIENTED_EDGE ( 'NONE', *, *, #2532, .T. ) ;
#12068=CARTESIAN_POINT ( 'NONE',  ( 4.898587196589413075E-17, 9.000000000000000000, 0.4000000000000000222 ) ) ;
#12069=( LENGTH_UNIT ( ) NAMED_UNIT ( * ) SI_UNIT ( .MILLI., .METRE. ) );
#12072=CARTESIAN_POINT ( 'NONE',  ( 8.481367827640703183, 0.000000000000000000, 0.5624942419805130100 ) ) ;
#12076=ORIENTED_EDGE ( 'NONE', *, *, #5186, .T. ) ;
#12082=VERTEX_POINT ( 'NONE', #12555 ) ;
#12083=DIRECTION ( 'NONE',  ( 0.000000000000000000, 0.000000000000000000, 1.000000000000000000 ) ) ;
#12089=CARTESIAN_POINT ( 'NONE',  ( -5.299649803506882861, 0.000000000000000000, -6.645578376649353913 ) ) ;
#12097=CIRCLE ( 'NONE', #10983, 8.500000000000000000 ) ;
#12098=ORIENTED_EDGE ( 'NONE', *, *, #9541, .F. ) ;
#12105=CARTESIAN_POINT ( 'NONE',  ( 5.053288777954493050, 9.000000000000000000, -4.475128213425755952 ) ) ;
#12121=CARTESIAN_POINT ( 'NONE',  ( -6.057461899949976747, 9.000000000000000000, 5.137313564148215939 ) ) ;
#12125=CIRCLE ( 'NONE', #3751, 0.4000000000000000222 ) ;
#12127=ORIENTED_EDGE ( 'NONE', *, *, #3953, .F. ) ;
#12134=AXIS2_PLACEMENT_3D ( 'NONE', #7471, #12849, #5262 ) ;
#12136=ORIENTED_EDGE ( 'NONE', *, *, #4287, .T. ) ;
#12138=DIRECTION ( 'NONE',  ( 0.000000000000000000, 0.000000000000000000, -1.000000000000000000 ) ) ;
#12141=FACE_OUTER_BOUND ( 'NONE', #5457, .T. ) ;
#12145=DIRECTION ( 'NONE',  ( -0.000000000000000000, -1.000000000000000000, -0.000000000000000000 ) ) ;
#12148=EDGE_LOOP ( 'NONE', ( #9172, #9969, #2855, #10394 ) ) ;
#12149=DIRECTION ( 'NONE',  ( -0.000000000000000000, -1.000000000000000000, -0.000000000000000000 ) ) ;
#12152=CARTESIAN_POINT ( 'NONE',  ( 5.053288777954493050, 9.000000000000000000, -4.475128213425755952 ) ) ;
#12163=CARTESIAN_POINT ( 'NONE',  ( 3.555260608155774271, 0.000000000000000000, 7.720759160088842776 ) ) ;
#12185=CARTESIAN_POINT ( 'NONE',  ( 0.000000000000000000, 9.000000000000000000, 0.000000000000000000 ) ) ;
#12201=CARTESIAN_POINT ( 'NONE',  ( -0.8973464813148227526, 9.000000000000000000, -7.308217849399443189 ) ) ;
#12208=CIRCLE ( 'NONE', #539, 8.499999999999996447 ) ;
#12212=CARTESIAN_POINT ( 'NONE',  ( 3.555260608155775159, 0.000000000000000000, 7.720759160088846329 ) ) ;
#12216=DIRECTION ( 'NONE',  ( 0.000000000000000000, 1.000000000000000000, -0.000000000000000000 ) ) ;
#12217=CARTESIAN_POINT ( 'NONE',  ( -5.526615004551211463, 9.000000000000000000, -4.866191470063547797 ) ) ;
#12228=DIRECTION ( 'NONE',  ( -0.000000000000000000, -1.000000000000000000, -0.000000000000000000 ) ) ;
#12237=DIRECTION ( 'NONE',  ( -0.000000000000000000, -1.000000000000000000, -0.000000000000000000 ) ) ;
#12242=ORIENTED_EDGE ( 'NONE', *, *, #2172, .T. ) ;
#12245=EDGE_LOOP ( 'NONE', ( #2223, #5456, #1386, #11979 ) ) ;
#12266=DIRECTION ( 'NONE',  ( 0.000000000000000000, 1.000000000000000000, -0.000000000000000000 ) ) ;
#12274=CARTESIAN_POINT ( 'NONE',  ( -1.604252589105052307, 0.000000000000000000, -8.347237484961700815 ) ) ;
#12276=CYLINDRICAL_SURFACE ( 'NONE', #3142, 8.499999999999998224 ) ;
#12278=ORIENTED_EDGE ( 'NONE', *, *, #6620, .T. ) ;
#12285=AXIS2_PLACEMENT_3D ( 'NONE', #3650, #2616, #11023 ) ;
#12288=CARTESIAN_POINT ( 'NONE',  ( 0.000000000000000000, 9.000000000000000000, 0.000000000000000000 ) ) ;
#12305=LINE ( 'NONE', #6777, #8801 ) ;
#12309=ORIENTED_EDGE ( 'NONE', *, *, #3952, .F. ) ;
#12315=EDGE_CURVE ( 'NONE', #10298, #12927, #2979, .T. ) ;
#12321=CARTESIAN_POINT ( 'NONE',  ( 5.958322434183388694, 0.000000000000000000, -6.062045345451230638 ) ) ;
#12324=CARTESIAN_POINT ( 'NONE',  ( 6.736042615721505200, 0.000000000000000000, 5.184180733653466433 ) ) ;
#12325=VERTEX_POINT ( 'NONE', #4957 ) ;
#12326=CARTESIAN_POINT ( 'NONE',  ( -7.751044794789887504, 0.000000000000000000, 1.733822342365972879 ) ) ;
#12327=CARTESIAN_POINT ( 'NONE',  ( 0.000000000000000000, 9.000000000000000000, 0.000000000000000000 ) ) ;
#12329=VERTEX_POINT ( 'NONE', #9154 ) ;
#12363=VERTEX_POINT ( 'NONE', #10947 ) ;
#12365=LINE ( 'NONE', #8206, #2245 ) ;
#12368=ADVANCED_FACE ( 'NONE', ( #5776 ), #4753, .T. ) ;
#12377=CIRCLE ( 'NONE', #6409, 8.500000000000000000 ) ;
#12380=CARTESIAN_POINT ( 'NONE',  ( -6.558450276537426404, 9.000000000000000000, -1.596630818375423866 ) ) ;
#12394=AXIS2_PLACEMENT_3D ( 'NONE', #2778, #4635, #6985 ) ;
#12399=B_SPLINE_SURFACE_WITH_KNOTS ( 'NONE', 3, 1, ( 
 ( #904, #9096 ),
 ( #8129, #2897 ),
 ( #9377, #13312 ),
 ( #5176, #13515 ) ),
 .UNSPECIFIED., .F., .F., .F.,
 ( 4, 4 ),
 ( 2, 2 ),
 ( 0.000000000000000000, 0.8724294488011768989 ),
 ( 0.000000000000000000, 1.000000000000000000 ),
 .UNSPECIFIED. ) ;
#12422=ORIENTED_EDGE ( 'NONE', *, *, #9036, .F. ) ;
#12424=ADVANCED_FACE ( 'NONE', ( #8054 ), #62, .T. ) ;
#12430=FACE_OUTER_BOUND ( 'NONE', #3795, .T. ) ;
#12431=DIRECTION ( 'NONE',  ( 0.000000000000000000, 0.000000000000000000, 1.000000000000000000 ) ) ;
#12433=FACE_OUTER_BOUND ( 'NONE', #2625, .T. ) ;
#12438=AXIS2_PLACEMENT_3D ( 'NONE', #12043, #5896, #8922 ) ;
#12440=VECTOR ( 'NONE', #1354, 1000.000000000000000 ) ;
#12441=CARTESIAN_POINT ( 'NONE',  ( 2.394769219159762041, 9.000000000000000000, -6.310909632292713844 ) ) ;
#12470=CARTESIAN_POINT ( 'NONE',  ( 0.000000000000000000, 0.000000000000000000, 0.000000000000000000 ) ) ;
#12473=CARTESIAN_POINT ( 'NONE',  ( -8.369528376005813897, 0.000000000000000000, 1.483574994138652903 ) ) ;
#12486=ORIENTED_EDGE ( 'NONE', *, *, #8352, .F. ) ;
#12490=EDGE_CURVE ( 'NONE', #1998, #11792, #9045, .T. ) ;
#12491=CARTESIAN_POINT ( 'NONE',  ( 0.000000000000000000, 9.000000000000000000, -0.4000000000000000222 ) ) ;
#12503=EDGE_LOOP ( 'NONE', ( #1965, #12596, #10067, #11499 ) ) ;
#12509=CARTESIAN_POINT ( 'NONE',  ( 2.623034112301249721, 9.000000000000000000, -7.496701717520498853 ) ) ;
#12520=ORIENTED_EDGE ( 'NONE', *, *, #510, .F. ) ;
#12523=ORIENTED_EDGE ( 'NONE', *, *, #9184, .F. ) ;
#12528=CARTESIAN_POINT ( 'NONE',  ( 6.554160776451332104, 1.734723475976807094E-15, -1.614148852004323231 ) ) ;
#12529=CARTESIAN_POINT ( 'NONE',  ( 0.000000000000000000, -3.000000000000000000, 0.000000000000000000 ) ) ;
#12535=CARTESIAN_POINT ( 'NONE',  ( -6.558450276537426404, 0.000000000000000000, -1.596630818375423866 ) ) ;
#12539=DIRECTION ( 'NONE',  ( 0.000000000000000000, 1.000000000000000000, -0.000000000000000000 ) ) ;
#12547=EDGE_LOOP ( 'NONE', ( #6781, #12064 ) ) ;
#12555=CARTESIAN_POINT ( 'NONE',  ( 8.481367827640703183, 9.000000000000000000, 0.5624942419805127880 ) ) ;
#12557=FACE_OUTER_BOUND ( 'NONE', #6385, .T. ) ;
#12571=LINE ( 'NONE', #2798, #6485 ) ;
#12574=CIRCLE ( 'NONE', #6617, 6.750000000000000888 ) ;
#12578=ORIENTED_EDGE ( 'NONE', *, *, #4287, .F. ) ;
#12589=EDGE_CURVE ( 'NONE', #1159, #6548, #8248, .T. ) ;
#12593=VECTOR ( 'NONE', #11585, 1000.000000000000000 ) ;
#12596=ORIENTED_EDGE ( 'NONE', *, *, #4654, .F. ) ;
#12601=CARTESIAN_POINT ( 'NONE',  ( 0.000000000000000000, 0.000000000000000000, 0.000000000000000000 ) ) ;
#12608=VECTOR ( 'NONE', #4613, 1000.000000000000000 ) ;
#12614=CARTESIAN_POINT ( 'NONE',  ( -6.515098946627274401, 0.000000000000000000, 3.430563300314522390 ) ) ;
#12621=CARTESIAN_POINT ( 'NONE',  ( -2.976187484161006314, 0.000000000000000000, 7.363908159724035229 ) ) ;
#12623=CIRCLE ( 'NONE', #2494, 9.250000000000000000 ) ;
#12625=CARTESIAN_POINT ( 'NONE',  ( -2.655466033450426533, 9.000000000000000000, -7.485541762018160128 ) ) ;
#12629=CARTESIAN_POINT ( 'NONE',  ( 0.000000000000000000, 0.000000000000000000, 0.000000000000000000 ) ) ;
#12630=ORIENTED_EDGE ( 'NONE', *, *, #11635, .F. ) ;
#12644=AXIS2_PLACEMENT_3D ( 'NONE', #4271, #4472, #8466 ) ;
#12645=VERTEX_POINT ( 'NONE', #4528 ) ;
#12647=ORIENTED_EDGE ( 'NONE', *, *, #6320, .F. ) ;
#12649=CARTESIAN_POINT ( 'NONE',  ( -7.235926821844430812, 9.000000000000000000, 4.459973433655439301 ) ) ;
#12652=EDGE_CURVE ( 'NONE', #1554, #10329, #12800, .T. ) ;
#12662=ORIENTED_EDGE ( 'NONE', *, *, #13491, .F. ) ;
#12665=DIRECTION ( 'NONE',  ( -0.000000000000000000, -1.000000000000000000, -0.000000000000000000 ) ) ;
#12670=LINE ( 'NONE', #7291, #13003 ) ;
#12673=EDGE_CURVE ( 'NONE', #7170, #13219, #12208, .T. ) ;
#12675=B_SPLINE_CURVE_WITH_KNOTS ( 'NONE', 3,
 ( #12321, #813, #2862, #7074 ),
 .UNSPECIFIED., .F., .F.,
 ( 4, 4 ),
 ( 0.1276832474596270861, 1.000000000000000000 ),
 .UNSPECIFIED. ) ;
#12696=ORIENTED_EDGE ( 'NONE', *, *, #2733, .F. ) ;
#12698=DIRECTION ( 'NONE',  ( 0.000000000000000000, 0.000000000000000000, 1.000000000000000000 ) ) ;
#12704=DIRECTION ( 'NONE',  ( -0.000000000000000000, -1.000000000000000000, -0.000000000000000000 ) ) ;
#12710=ORIENTED_EDGE ( 'NONE', *, *, #2119, .F. ) ;
#12722=CARTESIAN_POINT ( 'NONE',  ( 4.201465772524378472, 9.000000000000000000, 6.047394330962382547 ) ) ;
#12727=EDGE_CURVE ( 'NONE', #10584, #20, #759, .T. ) ;
#12733=B_SPLINE_CURVE_WITH_KNOTS ( 'NONE', 3,
 ( #6755, #9094, #13103, #6894 ),
 .UNSPECIFIED., .F., .F.,
 ( 4, 4 ),
 ( 0.1276832474596353850, 1.000000000000000000 ),
 .UNSPECIFIED. ) ;
#12739=DIRECTION ( 'NONE',  ( 0.000000000000000000, 1.000000000000000000, -0.000000000000000000 ) ) ;
#12745=CARTESIAN_POINT ( 'NONE',  ( -7.780961115628980629, 9.000000000000000000, -3.421497350147988392 ) ) ;
#12746=CARTESIAN_POINT ( 'NONE',  ( -6.558450276537426404, 0.000000000000000000, -1.596630818375420757 ) ) ;
#12756=CARTESIAN_POINT ( 'NONE',  ( -6.549210654805285081, 0.000000000000000000, 1.634117437329677180 ) ) ;
#12769=CARTESIAN_POINT ( 'NONE',  ( -8.369528376005813897, 0.000000000000000000, 1.483574994138652903 ) ) ;
#12777=CARTESIAN_POINT ( 'NONE',  ( -0.4399887592034530392, 9.000000000000000000, 8.488604708182295511 ) ) ;
#12779=CARTESIAN_POINT ( 'NONE',  ( -6.549210654805285969, 0.000000000000000000, 1.634117437329680067 ) ) ;
#12780=CIRCLE ( 'NONE', #5960, 6.749999999999999112 ) ;
#12800=LINE ( 'NONE', #3221, #4964 ) ;
#12802=VERTEX_POINT ( 'NONE', #3624 ) ;
#12803=ORIENTED_EDGE ( 'NONE', *, *, #11345, .F. ) ;
#12810=EDGE_CURVE ( 'NONE', #1004, #7453, #7824, .T. ) ;
#12813=CARTESIAN_POINT ( 'NONE',  ( 2.620242232815953809, 0.000000000000000000, 6.881105251569436199 ) ) ;
#12817=VECTOR ( 'NONE', #12987, 1000.000000000000000 ) ;
#12820=ORIENTED_EDGE ( 'NONE', *, *, #321, .F. ) ;
#12824=ORIENTED_EDGE ( 'NONE', *, *, #24, .F. ) ;
#12826=CARTESIAN_POINT ( 'NONE',  ( 0.000000000000000000, -3.000000000000000000, 9.250000000000000000 ) ) ;
#12830=SURFACE_SIDE_STYLE ('',( #6622 ) ) ;
#12837=CARTESIAN_POINT ( 'NONE',  ( -0.4399887592034473771, 9.000000000000000000, 8.488604708182295511 ) ) ;
#12849=DIRECTION ( 'NONE',  ( 0.000000000000000000, 1.000000000000000000, -0.000000000000000000 ) ) ;
#12867=CARTESIAN_POINT ( 'NONE',  ( 0.000000000000000000, 9.000000000000000000, 0.000000000000000000 ) ) ;
#12880=DIRECTION ( 'NONE',  ( 0.000000000000000000, 0.000000000000000000, 1.000000000000000000 ) ) ;
#12886=DIRECTION ( 'NONE',  ( 0.000000000000000000, -1.000000000000000000, 0.000000000000000000 ) ) ;
#12888=CARTESIAN_POINT ( 'NONE',  ( -2.590203375110137873, 0.000000000000000000, 6.893050072893555758 ) ) ;
#12890=ORIENTED_EDGE ( 'NONE', *, *, #3263, .T. ) ;
#12903=DIRECTION ( 'NONE',  ( -0.000000000000000000, -1.000000000000000000, -0.000000000000000000 ) ) ;
#12912=EDGE_CURVE ( 'NONE', #479, #6815, #8660, .T. ) ;
#12917=CARTESIAN_POINT ( 'NONE',  ( -7.363095878837111030, 9.000000000000000000, 0.009895496992605581216 ) ) ;
#12924=CARTESIAN_POINT ( 'NONE',  ( 0.000000000000000000, 0.000000000000000000, -6.750000000000000888 ) ) ;
#12927=VERTEX_POINT ( 'NONE', #12990 ) ;
#12942=ORIENTED_EDGE ( 'NONE', *, *, #108, .F. ) ;
#12945=CARTESIAN_POINT ( 'NONE',  ( 0.000000000000000000, 9.000000000000000000, 0.000000000000000000 ) ) ;
#12953=B_SPLINE_CURVE_WITH_KNOTS ( 'NONE', 3,
 ( #9021, #10065, #13032, #635 ),
 .UNSPECIFIED., .F., .F.,
 ( 4, 4 ),
 ( 0.1276832474596256706, 1.000000000000000000 ),
 .UNSPECIFIED. ) ;
#12956=ORIENTED_EDGE ( 'NONE', *, *, #2793, .F. ) ;
#12969=ORIENTED_EDGE ( 'NONE', *, *, #1555, .T. ) ;
#12973=CARTESIAN_POINT ( 'NONE',  ( 5.985774866078160450, 9.000000000000000000, 3.119775513178307147 ) ) ;
#12980=DIRECTION ( 'NONE',  ( 0.000000000000000000, 0.000000000000000000, 1.000000000000000000 ) ) ;
#12987=DIRECTION ( 'NONE',  ( -0.000000000000000000, -1.000000000000000000, -0.000000000000000000 ) ) ;
#12990=CARTESIAN_POINT ( 'NONE',  ( 5.280889752749253319, 9.000000000000000000, -6.660495733750448011 ) ) ;
#12994=EDGE_CURVE ( 'NONE', #12802, #710, #1643, .T. ) ;
#12995=CARTESIAN_POINT ( 'NONE',  ( 3.818534268238711338, 9.000000000000000000, -5.566084444408533116 ) ) ;
#12999=DIRECTION ( 'NONE',  ( 0.000000000000000000, 0.000000000000000000, -1.000000000000000000 ) ) ;
#13003=VECTOR ( 'NONE', #7486, 1000.000000000000000 ) ;
#13005=VERTEX_POINT ( 'NONE', #9950 ) ;
#13026=CARTESIAN_POINT ( 'NONE',  ( 0.000000000000000000, 0.000000000000000000, 0.000000000000000000 ) ) ;
#13027=DIRECTION ( 'NONE',  ( 0.000000000000000000, 0.000000000000000000, -1.000000000000000000 ) ) ;
#13032=CARTESIAN_POINT ( 'NONE',  ( -0.8776997859584816375, 0.000000000000000000, 7.310603390113379341 ) ) ;
#13033=CARTESIAN_POINT ( 'NONE',  ( -0.8123631076467130452, 9.000000000000000000, -6.700937709107179785 ) ) ;
#13046=CARTESIAN_POINT ( 'NONE',  ( 6.530577460941774603, 0.000000000000000000, 3.402183248810843885 ) ) ;
#13049=CARTESIAN_POINT ( 'NONE',  ( -7.363095878837111030, 0.000000000000000000, 0.009895496992605581216 ) ) ;
#13051=DIRECTION ( 'NONE',  ( 0.000000000000000000, 1.000000000000000000, -0.000000000000000000 ) ) ;
#13052=CARTESIAN_POINT ( 'NONE',  ( 0.8327827707325454742, 0.000000000000000000, 6.698430626405788679 ) ) ;
#13056=ORIENTED_EDGE ( 'NONE', *, *, #5633, .T. ) ;
#13064=DIRECTION ( 'NONE',  ( -0.000000000000000000, -1.000000000000000000, -0.000000000000000000 ) ) ;
#13066=FACE_OUTER_BOUND ( 'NONE', #7651, .T. ) ;
#13074=EDGE_LOOP ( 'NONE', ( #4669, #6275, #6576, #10343 ) ) ;
#13075=AXIS2_PLACEMENT_3D ( 'NONE', #13176, #9804, #10075 ) ;
#13084=DIRECTION ( 'NONE',  ( 0.000000000000000000, 0.000000000000000000, -1.000000000000000000 ) ) ;
#13088=DIRECTION ( 'NONE',  ( 0.000000000000000000, 1.000000000000000000, -0.000000000000000000 ) ) ;
#13101=CARTESIAN_POINT ( 'NONE',  ( 0.8653219153705552502, 9.000000000000000000, -7.312626806738413698 ) ) ;
#13102=( NAMED_UNIT ( * ) PLANE_ANGLE_UNIT ( ) SI_UNIT ( $, .RADIAN. ) );
#13103=CARTESIAN_POINT ( 'NONE',  ( -6.515098946627274401, -1.694065894508600678E-18, 3.430563300314522390 ) ) ;
#13117=FACE_OUTER_BOUND ( 'NONE', #3505, .T. ) ;
#13167=DIRECTION ( 'NONE',  ( -0.000000000000000000, -1.000000000000000000, -0.000000000000000000 ) ) ;
#13176=CARTESIAN_POINT ( 'NONE',  ( 0.000000000000000000, 0.000000000000000000, 0.000000000000000000 ) ) ;
#13190=VECTOR ( 'NONE', #11286, 1000.000000000000000 ) ;
#13191=ORIENTED_EDGE ( 'NONE', *, *, #10280, .F. ) ;
#13208=EDGE_LOOP ( 'NONE', ( #9940, #1869, #3354, #1461 ) ) ;
#13210=CARTESIAN_POINT ( 'NONE',  ( 0.000000000000000000, 0.000000000000000000, 0.000000000000000000 ) ) ;
#13213=CARTESIAN_POINT ( 'NONE',  ( -0.8973464813148227526, -1.694065894508600678E-18, -7.308217849399443189 ) ) ;
#13215=VECTOR ( 'NONE', #1353, 1000.000000000000000 ) ;
#13219=VERTEX_POINT ( 'NONE', #4304 ) ;
#13223=CARTESIAN_POINT ( 'NONE',  ( -2.976187484161006314, 9.000000000000000000, 7.363908159724035229 ) ) ;
#13231=DIRECTION ( 'NONE',  ( -0.000000000000000000, -1.000000000000000000, -0.000000000000000000 ) ) ;
#13255=CARTESIAN_POINT ( 'NONE',  ( -5.299649803506882861, 9.000000000000000000, -6.645578376649353913 ) ) ;
#13257=EDGE_CURVE ( 'NONE', #5342, #8278, #7228, .T. ) ;
#13259=CARTESIAN_POINT ( 'NONE',  ( 0.000000000000000000, 0.000000000000000000, 0.000000000000000000 ) ) ;
#13280=ORIENTED_EDGE ( 'NONE', *, *, #12912, .T. ) ;
#13284=DIRECTION ( 'NONE',  ( 0.000000000000000000, 1.000000000000000000, -0.000000000000000000 ) ) ;
#13286=CIRCLE ( 'NONE', #7537, 8.500000000000001776 ) ;
#13302=DIRECTION ( 'NONE',  ( 0.000000000000000000, 0.000000000000000000, 1.000000000000000000 ) ) ;
#13303=ORIENTED_EDGE ( 'NONE', *, *, #3026, .F. ) ;
#13312=CARTESIAN_POINT ( 'NONE',  ( -2.976187484161006314, 0.000000000000000000, 7.363908159724035229 ) ) ;
#13324=ORIENTED_EDGE ( 'NONE', *, *, #7064, .F. ) ;
#13332=DIRECTION ( 'NONE',  ( 0.000000000000000000, 1.000000000000000000, -0.000000000000000000 ) ) ;
#13334=CARTESIAN_POINT ( 'NONE',  ( -3.833392836528145331, 9.000000000000000000, -5.555861711818853799 ) ) ;
#13339=CARTESIAN_POINT ( 'NONE',  ( -7.939678587550617728, 9.000000000000000000, 0.2057875656132798770 ) ) ;
#13348=B_SPLINE_CURVE_WITH_KNOTS ( 'NONE', 3,
 ( #1509, #3638, #8938, #8790 ),
 .UNSPECIFIED., .F., .F.,
 ( 4, 4 ),
 ( 0.000000000000000000, 0.8724294488011762327 ),
 .UNSPECIFIED. ) ;
#13353=EDGE_CURVE ( 'NONE', #3503, #8945, #1873, .T. ) ;
#13356=CARTESIAN_POINT ( 'NONE',  ( -6.549210654805285081, 0.000000000000000000, 1.634117437329677180 ) ) ;
#13364=CARTESIAN_POINT ( 'NONE',  ( 0.000000000000000000, 0.000000000000000000, 0.000000000000000000 ) ) ;
#13372=CARTESIAN_POINT ( 'NONE',  ( 0.000000000000000000, 0.000000000000000000, 0.000000000000000000 ) ) ;
#13374=ORIENTED_EDGE ( 'NONE', *, *, #5677, .F. ) ;
#13381=CARTESIAN_POINT ( 'NONE',  ( 0.7944557581062194895, 0.000000000000000000, -6.703084368289861317 ) ) ;
#13389=B_SPLINE_CURVE_WITH_KNOTS ( 'NONE', 3,
 ( #6141, #2147, #984, #10490 ),
 .UNSPECIFIED., .F., .F.,
 ( 4, 4 ),
 ( 0.1276832474596253097, 1.000000000000000000 ),
 .UNSPECIFIED. ) ;
#13397=CARTESIAN_POINT ( 'NONE',  ( -4.174571361198896824, 0.000000000000000000, 6.065330394303907191 ) ) ;
#13400=ORIENTED_EDGE ( 'NONE', *, *, #8352, .T. ) ;
#13416=MANIFOLD_SOLID_BREP ( 'Boss-Extrude2', #5104 ) ;
#13419=EDGE_LOOP ( 'NONE', ( #8303, #5052 ) ) ;
#13451=CARTESIAN_POINT ( 'NONE',  ( -2.411622991978543684, 9.000000000000000000, -6.304488444319686913 ) ) ;
#13456=VECTOR ( 'NONE', #591, 1000.000000000000000 ) ;
#13485=DIRECTION ( 'NONE',  ( -0.000000000000000000, -1.000000000000000000, -0.000000000000000000 ) ) ;
#13491=EDGE_CURVE ( 'NONE', #8876, #3254, #9516, .T. ) ;
#13493=CARTESIAN_POINT ( 'NONE',  ( 0.000000000000000000, 9.000000000000000000, 0.000000000000000000 ) ) ;
#13501=DIRECTION ( 'NONE',  ( 0.000000000000000000, 0.000000000000000000, 1.000000000000000000 ) ) ;
#13508=ORIENTED_EDGE ( 'NONE', *, *, #2402, .T. ) ;
#13515=CARTESIAN_POINT ( 'NONE',  ( -3.533475733155563070, 0.000000000000000000, 7.730753471893976325 ) ) ;
#13522=ORIENTED_EDGE ( 'NONE', *, *, #460, .F. ) ;
#13525=ORIENTED_EDGE ( 'NONE', *, *, #12490, .T. ) ;
#13536=CARTESIAN_POINT ( 'NONE',  ( 2.458659560121116527, 0.000000000000000000, -8.136645080586040635 ) ) ;
#13539=AXIS2_PLACEMENT_3D ( 'NONE', #7317, #9715, #3106 ) ;
#13541=DIRECTION ( 'NONE',  ( -0.000000000000000000, -1.000000000000000000, -0.000000000000000000 ) ) ;
#13555=DIRECTION ( 'NONE',  ( 0.000000000000000000, -1.000000000000000000, 0.000000000000000000 ) ) ;
#13558=B_SPLINE_SURFACE_WITH_KNOTS ( 'NONE', 3, 1, ( 
 ( #2493, #421 ),
 ( #1466, #5653 ),
 ( #4132, #1940 ),
 ( #5928, #2972 ) ),
 .UNSPECIFIED., .F., .F., .F.,
 ( 4, 4 ),
 ( 2, 2 ),
 ( 0.000000000000000000, 0.8724294488011784532 ),
 ( 0.000000000000000000, 1.000000000000000000 ),
 .UNSPECIFIED. ) ;
#13565=CARTESIAN_POINT ( 'NONE',  ( -3.833392836528144443, 9.000000000000000000, -5.555861711818853799 ) ) ;
#13567=CARTESIAN_POINT ( 'NONE',  ( 5.517918333394296049, 9.000000000000000000, 4.875228826198821253 ) ) ;
#13579=CARTESIAN_POINT ( 'NONE',  ( -5.065227977808753224, 9.000000000000000000, -4.461610195077944319 ) ) ;
#13589=AXIS2_PLACEMENT_3D ( 'NONE', #7850, #4554, #12138 ) ;
#13595=FACE_OUTER_BOUND ( 'NONE', #10965, .T. ) ;
#13622=COLOUR_RGB('Dark Blue',0.08,0.2,0.34);
#13623=FILL_AREA_STYLE_COLOUR('',#13622);
#13624=FILL_AREA_STYLE('',(#13623));
#13625=SURFACE_STYLE_FILL_AREA(#13624);
#13626=SURFACE_SIDE_STYLE('',(#13625));
#13627=SURFACE_STYLE_USAGE(.BOTH.,#13626);
#13628=PRESENTATION_STYLE_ASSIGNMENT((#13627));
ENDSEC;
END-ISO-10303-21;
